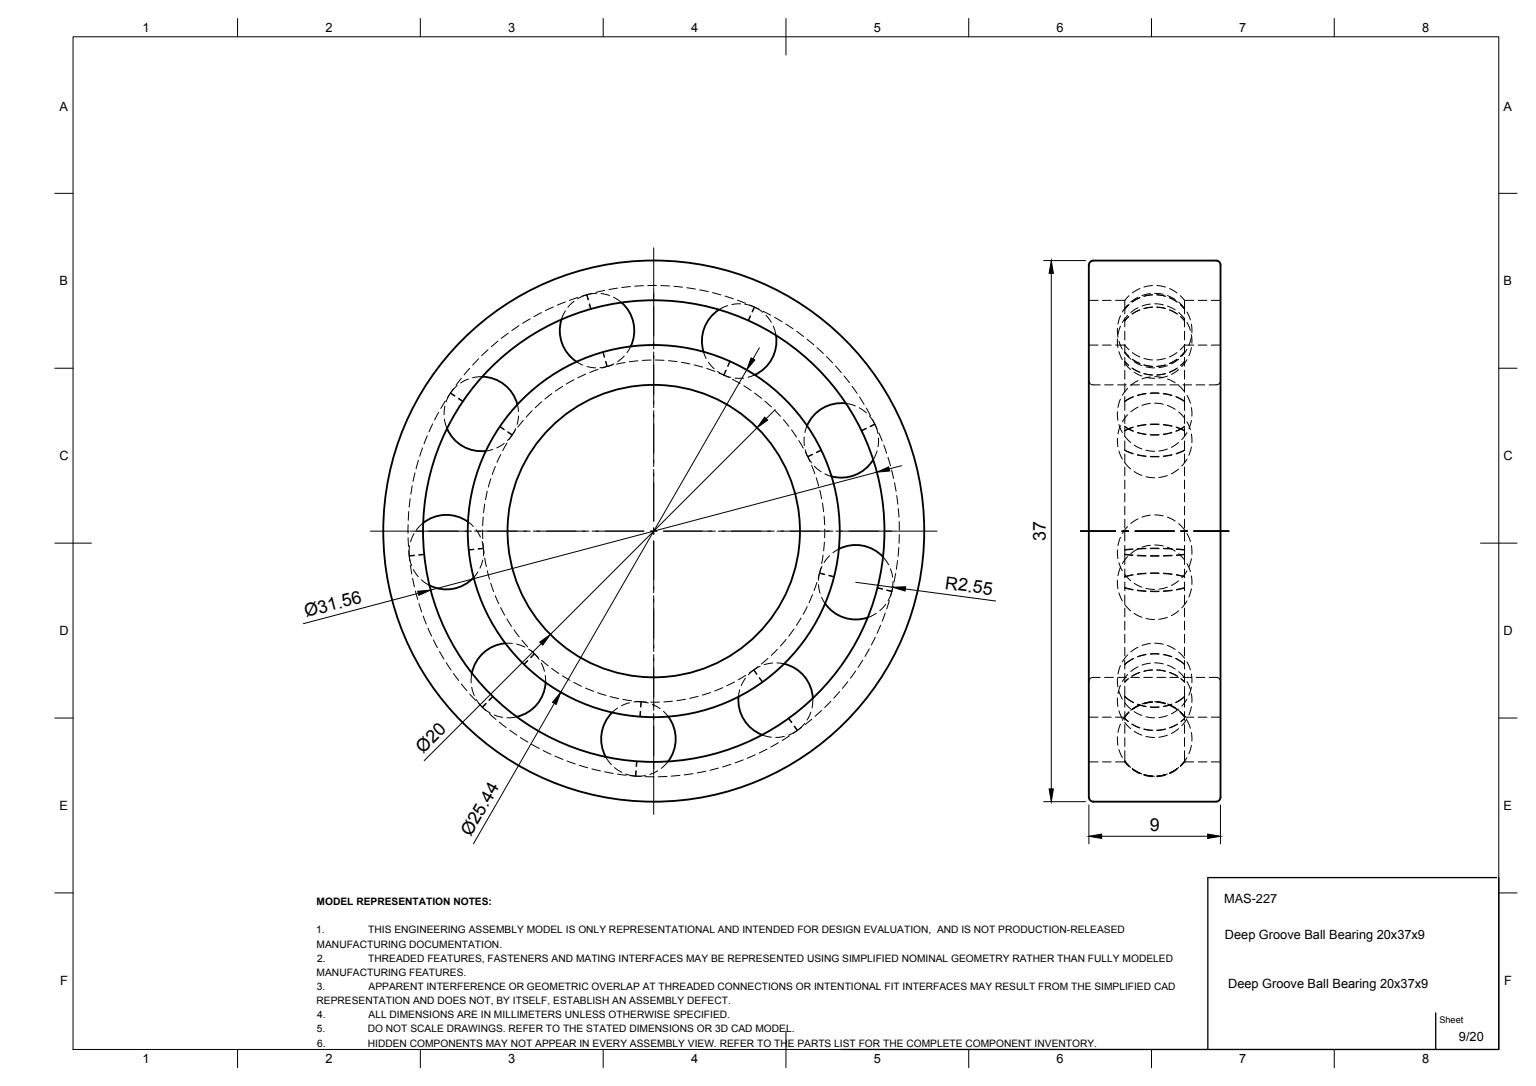
ISO-10303-21;
HEADER;
FILE_DESCRIPTION (('STEP AP214'),
    '1' );
FILE_NAME ( 'Deep Groove Ball Bearing 20x37x9.step', '2026-10-06T08:24:41', ( '' ), ( '' ), 'STEP AP214', 'Unspecified', '' );
FILE_SCHEMA (( 'AUTOMOTIVE_DESIGN' ));
ENDSEC;
DATA;
#3=CARTESIAN_POINT ( 'NONE',  ( -0.4535326485287288212, 0.08054850140359781641, 0.1903859677775356918 ) ) ;
#22=ORIENTED_EDGE ( 'NONE', *, *, #12287, .T. ) ;
#27=ORIENTED_EDGE ( 'NONE', *, *, #23684, .F. ) ;
#29=ORIENTED_EDGE ( 'NONE', *, *, #17755, .F. ) ;
#40=CARTESIAN_POINT ( 'NONE',  ( -2.184900367198595585E-17, 0.6212598425196850238, 0.2574827755769818483 ) ) ;
#60=CARTESIAN_POINT ( 'NONE',  ( -0.4335958738490826581, -0.2505647196907692664, 0.09684793308443542803 ) ) ;
#63=ADVANCED_FACE ( 'NONE', ( #7520 ), #26320, .F. ) ;
#85=ORIENTED_EDGE ( 'NONE', *, *, #20703, .F. ) ;
#95=CARTESIAN_POINT ( 'NONE',  ( 0.1709077104829875848, -0.4707213777573787672, 0.09684874903502814492 ) ) ;
#98=CARTESIAN_POINT ( 'NONE',  ( -0.4055118110236220486, 4.966087413865251393E-17, 0.3543307086614173040 ) ) ;
#129=EDGE_CURVE ( 'NONE', #7282, #11900, #2406, .T. ) ;
#130=TOROIDAL_SURFACE ( 'NONE', #25799, 0.5610236220472440971, 0.1003937007874015908 ) ;
#131=DIRECTION ( 'NONE',  ( 0.000000000000000000, 0.000000000000000000, -1.000000000000000000 ) ) ;
#139=DIRECTION ( 'NONE',  ( 0.000000000000000000, 0.000000000000000000, 1.000000000000000000 ) ) ;
#140=ORIENTED_EDGE ( 'NONE', *, *, #5854, .T. ) ;
#145=ORIENTED_EDGE ( 'NONE', *, *, #17289, .F. ) ;
#146=CARTESIAN_POINT ( 'NONE',  ( -2.183966630091013010E-17, 0.6212598425196852459, 0.09684793308443542803 ) ) ;
#160=DIRECTION ( 'NONE',  ( 0.000000000000000000, 0.000000000000000000, 1.000000000000000000 ) ) ;
#168=CARTESIAN_POINT ( 'NONE',  ( -0.2120693917185543231, -0.5839438448129543602, 0.09684874924366436433 ) ) ;
#180=ORIENTED_EDGE ( 'NONE', *, *, #22193, .F. ) ;
#184=CARTESIAN_POINT ( 'NONE',  ( 0.4932478747986535628, 0.08657132889677619791, 0.09684874903502814492 ) ) ;
#195=CARTESIAN_POINT ( 'NONE',  ( 0.000000000000000000, 0.000000000000000000, -3.278217716535432842E-17 ) ) ;
#198=CARTESIAN_POINT ( 'NONE',  ( -0.1709077104829878069, -0.4707213777573787672, 0.09684874903502814492 ) ) ;
#204=CIRCLE ( 'NONE', #17722, 0.6212598425196850238 ) ;
#210=CIRCLE ( 'NONE', #27230, 0.6212598425196850238 ) ;
#220=CARTESIAN_POINT ( 'NONE',  ( 0.000000000000000000, 0.000000000000000000, 0.1771653543307086520 ) ) ;
#221=EDGE_LOOP ( 'NONE', ( #12338, #6881, #25054, #27642 ) ) ;
#225=CIRCLE ( 'NONE', #16892, 0.5007874015748031704 ) ;
#233=EDGE_CURVE ( 'NONE', #14152, #23049, #22735, .T. ) ;
#248=CARTESIAN_POINT ( 'NONE',  ( 0.3998447049182889956, 0.4754871227240441423, 0.2574803149606298969 ) ) ;
#261=CARTESIAN_POINT ( 'NONE',  ( 0.2965233727166233790, 0.3524965443697388734, 0.1771653543307087630 ) ) ;
#274=ORIENTED_EDGE ( 'NONE', *, *, #6413, .T. ) ;
#279=DIRECTION ( 'NONE',  ( 0.000000000000000000, 1.000000000000000000, 0.000000000000000000 ) ) ;
#290=VERTEX_POINT ( 'NONE', #22923 ) ;
#300=ADVANCED_FACE ( 'NONE', ( #3258 ), #20928, .T. ) ;
#316=ORIENTED_EDGE ( 'NONE', *, *, #13974, .F. ) ;
#318=ORIENTED_EDGE ( 'NONE', *, *, #26206, .F. ) ;
#323=CARTESIAN_POINT ( 'NONE',  ( -0.4126915023524561632, -0.2375990495015092296, 0.2330651858026694390 ) ) ;
#325=CARTESIAN_POINT ( 'NONE',  ( -0.1716509673353403542, -0.4704508543867079173, 0.09684874903502814492 ) ) ;
#327=CARTESIAN_POINT ( 'NONE',  ( 0.5692936381926190226, -0.3294684677443725507, 0.2081850588275903358 ) ) ;
#328=FACE_OUTER_BOUND ( 'NONE', #1258, .T. ) ;
#342=CARTESIAN_POINT ( 'NONE',  ( -0.4333973147258542991, -0.2509079296564011852, 0.09685039370078740717 ) ) ;
#344=ADVANCED_FACE ( 'NONE', ( #1581, #10184 ), #10334, .T. ) ;
#354=CARTESIAN_POINT ( 'NONE',  ( 0.1718374205099799101, -0.4703827404237102550, 0.09685039370078740717 ) ) ;
#377=LINE ( 'NONE', #8956, #9112 ) ;
#393=DIRECTION ( 'NONE',  ( 0.6427876096865396960, 0.7660444431189776804, -0.000000000000000000 ) ) ;
#407=ORIENTED_EDGE ( 'NONE', *, *, #26451, .F. ) ;
#424=CARTESIAN_POINT ( 'NONE',  ( -0.3991696156513551141, 0.4760540497243913594, 0.09684793308443542803 ) ) ;
#437=EDGE_LOOP ( 'NONE', ( #11123, #6651, #25287, #3751, #12023, #11943, #16300, #8034, #5039, #15886, #22940, #20148, #24795, #15480 ) ) ;
#442=ORIENTED_EDGE ( 'NONE', *, *, #8042, .F. ) ;
#448=DIRECTION ( 'NONE',  ( 0.000000000000000000, 1.000000000000000000, 0.000000000000000000 ) ) ;
#450=DIRECTION ( 'NONE',  ( 0.000000000000000000, 0.000000000000000000, 1.000000000000000000 ) ) ;
#454=DIRECTION ( 'NONE',  ( -0.9396926207859082059, 0.3420201433256690460, 0.000000000000000000 ) ) ;
#466=ORIENTED_EDGE ( 'NONE', *, *, #18480, .T. ) ;
#471=DIRECTION ( 'NONE',  ( -0.9848077530122080203, 0.1736481776669311083, 0.000000000000000000 ) ) ;
#473=DIRECTION ( 'NONE',  ( 0.000000000000000000, 0.000000000000000000, 1.000000000000000000 ) ) ;
#474=CARTESIAN_POINT ( 'NONE',  ( 0.1710938124795997883, -0.4706537664821763833, 0.09684793308443542803 ) ) ;
#478=VERTEX_POINT ( 'NONE', #6529 ) ;
#488=ORIENTED_EDGE ( 'NONE', *, *, #21767, .T. ) ;
#505=CARTESIAN_POINT ( 'NONE',  ( 0.6512499169092683671, 0.1155267097728963771, 0.1926811207759472899 ) ) ;
#512=ORIENTED_EDGE ( 'NONE', *, *, #14893, .F. ) ;
#547=CARTESIAN_POINT ( 'NONE',  ( -0.4210617728863489950, -0.2437762437896736079, 0.2467937633087636806 ) ) ;
#553=CARTESIAN_POINT ( 'NONE',  ( -0.2956505864974144360, 0.3532288989643737054, 0.1903859677777559323 ) ) ;
#564=AXIS2_PLACEMENT_3D ( 'NONE', #14105, #3204, #1666 ) ;
#566=DIRECTION ( 'NONE',  ( 0.000000000000000000, 0.000000000000000000, 1.000000000000000000 ) ) ;
#568=CARTESIAN_POINT ( 'NONE',  ( -0.1669561253487713837, -0.4569961989594632512, 0.2467937633337932146 ) ) ;
#580=ADVANCED_FACE ( 'NONE', ( #26282 ), #25912, .F. ) ;
#588=EDGE_CURVE ( 'NONE', #1674, #11878, #12352, .T. ) ;
#590=DIRECTION ( 'NONE',  ( -1.000000000000000000, 1.224646799147346305E-16, 0.000000000000000000 ) ) ;
#595=ADVANCED_FACE ( 'NONE', ( #719 ), #17319, .T. ) ;
#621=CARTESIAN_POINT ( 'NONE',  ( -0.5383572925356228112, -0.3100567972183445042, 0.2574803149606298969 ) ) ;
#625=FACE_OUTER_BOUND ( 'NONE', #9890, .T. ) ;
#639=DIRECTION ( 'NONE',  ( 0.000000000000000000, 0.000000000000000000, 1.000000000000000000 ) ) ;
#640=ORIENTED_EDGE ( 'NONE', *, *, #8614, .T. ) ;
#659=CARTESIAN_POINT ( 'NONE',  ( 0.6119360453657125554, 0.1072290460171897442, 0.09685039370078740717 ) ) ;
#692=ORIENTED_EDGE ( 'NONE', *, *, #26206, .T. ) ;
#693=CARTESIAN_POINT ( 'NONE',  ( 0.000000000000000000, 0.000000000000000000, 0.3425196850393700809 ) ) ;
#702=CARTESIAN_POINT ( 'NONE',  ( -0.0005939837304750000086, 0.5007870493127504208, 0.2574803149606298969 ) ) ;
#705=EDGE_CURVE ( 'NONE', #13715, #9472, #19846, .T. ) ;
#719=FACE_OUTER_BOUND ( 'NONE', #2456, .T. ) ;
#730=VERTEX_POINT ( 'NONE', #18485 ) ;
#731=DIRECTION ( 'NONE',  ( 0.000000000000000000, 1.000000000000000000, 0.000000000000000000 ) ) ;
#746=EDGE_CURVE ( 'NONE', #25825, #26393, #21042, .T. ) ;
#747=CARTESIAN_POINT ( 'NONE',  ( 0.6117833106356003192, 0.1080972763116094665, 0.2574827755769819038 ) ) ;
#753=TOROIDAL_SURFACE ( 'NONE', #16532, 0.7165354330708662012, 0.01181102362204724393 ) ;
#760=B_SPLINE_CURVE_WITH_KNOTS ( 'NONE', 3,
 ( #11709, #11429, #14120, #13834, #3353, #22726 ),
 .UNSPECIFIED., .F., .F.,
 ( 4, 2, 4 ),
 ( 0.9031406754215589583, 0.9046454396443730506, 0.9061502038671870318 ),
 .UNSPECIFIED. ) ;
#761=CARTESIAN_POINT ( 'NONE',  ( -7.608238775805210269E-17, -0.6212598425196850238, 0.3059055118110236560 ) ) ;
#765=EDGE_CURVE ( 'NONE', #26553, #20265, #18689, .T. ) ;
#769=CARTESIAN_POINT ( 'NONE',  ( -0.4931105264837953306, 0.08735026989778622852, 0.09684874903502814492 ) ) ;
#772=CARTESIAN_POINT ( 'NONE',  ( 0.000000000000000000, 0.000000000000000000, 0.3425196850393700809 ) ) ;
#776=DIRECTION ( 'NONE',  ( 0.000000000000000000, 0.000000000000000000, 1.000000000000000000 ) ) ;
#777=MECHANICAL_DESIGN_GEOMETRIC_PRESENTATION_REPRESENTATION('',(#15229),#16556);
#798=VERTEX_POINT ( 'NONE', #6495 ) ;
#811=DIRECTION ( 'NONE',  ( 0.000000000000000000, 1.000000000000000000, 0.000000000000000000 ) ) ;
#818=CARTESIAN_POINT ( 'NONE',  ( 0.6117062799105531523, 0.1085321106658064944, 0.2574803149606298969 ) ) ;
#829=CARTESIAN_POINT ( 'NONE',  ( 0.4121125639445893385, -0.2386018002037871011, 0.1212655228849990885 ) ) ;
#832=CARTESIAN_POINT ( 'NONE',  ( 0.2118615749922464486, -0.5840192333899535404, 0.2574803149606298969 ) ) ;
#833=VERTEX_POINT ( 'NONE', #19057 ) ;
#852=DIRECTION ( 'NONE',  ( 0.000000000000000000, 1.000000000000000000, 0.000000000000000000 ) ) ;
#882=CARTESIAN_POINT ( 'NONE',  ( -0.2255758929758618081, -0.6217623271429643106, 0.1616495878894404215 ) ) ;
#887=CARTESIAN_POINT ( 'NONE',  ( -0.4931450244001936989, 0.08715529520342381320, 0.2574827755769819038 ) ) ;
#897=FACE_OUTER_BOUND ( 'NONE', #27032, .T. ) ;
#900=CARTESIAN_POINT ( 'NONE',  ( -0.3998447049182095037, 0.4754871227241110332, 0.2574803149606298969 ) ) ;
#941=ORIENTED_EDGE ( 'NONE', *, *, #17711, .F. ) ;
#958=CARTESIAN_POINT ( 'NONE',  ( 0.000000000000000000, 0.000000000000000000, -3.278217716535432842E-17 ) ) ;
#969=EDGE_CURVE ( 'NONE', #16082, #26393, #16448, .T. ) ;
#973=CARTESIAN_POINT ( 'NONE',  ( 0.2243259791921815294, -0.6183223858027685482, 0.2081850588255441115 ) ) ;
#980=ORIENTED_EDGE ( 'NONE', *, *, #22815, .T. ) ;
#982=ORIENTED_EDGE ( 'NONE', *, *, #7627, .T. ) ;
#1008=CARTESIAN_POINT ( 'NONE',  ( -0.3223547283257516272, 0.3832433309296771617, 0.09685039370078740717 ) ) ;
#1013=ORIENTED_EDGE ( 'NONE', *, *, #10554, .F. ) ;
#1015=DIRECTION ( 'NONE',  ( 1.000000000000000000, 0.000000000000000000, 0.000000000000000000 ) ) ;
#1022=ORIENTED_EDGE ( 'NONE', *, *, #21337, .F. ) ;
#1026=ADVANCED_FACE ( 'NONE', ( #5184 ), #7886, .F. ) ;
#1040=CARTESIAN_POINT ( 'NONE',  ( 0.1707210962531913734, -0.4707890492249701131, 0.2574803149606298969 ) ) ;
#1042=CARTESIAN_POINT ( 'NONE',  ( 0.3998447049182889956, 0.4754871227240441423, 0.2574803149606298969 ) ) ;
#1044=DIRECTION ( 'NONE',  ( 1.000000000000000000, 0.000000000000000000, 0.000000000000000000 ) ) ;
#1057=DIRECTION ( 'NONE',  ( 0.000000000000000000, 0.000000000000000000, -1.000000000000000000 ) ) ;
#1074=DIRECTION ( 'NONE',  ( 0.000000000000000000, 0.000000000000000000, 1.000000000000000000 ) ) ;
#1079=ORIENTED_EDGE ( 'NONE', *, *, #19204, .T. ) ;
#1101=EDGE_CURVE ( 'NONE', #17070, #17929, #9204, .T. ) ;
#1110=DIRECTION ( 'NONE',  ( -0.8660254037844385966, -0.5000000000000002220, 0.000000000000000000 ) ) ;
#1116=CARTESIAN_POINT ( 'NONE',  ( 0.1589886963209722337, -0.4351482077926094871, 0.1494804571181609920 ) ) ;
#1126=EDGE_LOOP ( 'NONE', ( #5710, #17595 ) ) ;
#1132=EDGE_CURVE ( 'NONE', #24679, #11735, #20131, .T. ) ;
#1165=VERTEX_POINT ( 'NONE', #5771 ) ;
#1167=ORIENTED_EDGE ( 'NONE', *, *, #24794, .F. ) ;
#1175=ORIENTED_EDGE ( 'NONE', *, *, #10870, .F. ) ;
#1180=FACE_OUTER_BOUND ( 'NONE', #1413, .T. ) ;
#1185=ORIENTED_EDGE ( 'NONE', *, *, #7200, .F. ) ;
#1193=ORIENTED_EDGE ( 'NONE', *, *, #9457, .F. ) ;
#1195=DIRECTION ( 'NONE',  ( 0.000000000000000000, 0.000000000000000000, 1.000000000000000000 ) ) ;
#1205=VECTOR ( 'NONE', #24148, 39.37007874015748143 ) ;
#1224=EDGE_LOOP ( 'NONE', ( #22539, #14658 ) ) ;
#1229=B_SPLINE_CURVE_WITH_KNOTS ( 'NONE', 3,
 ( #14885, #198, #17116, #11030, #325, #8767 ),
 .UNSPECIFIED., .F., .F.,
 ( 4, 2, 4 ),
 ( 0.3000437156586439613, 0.3015484798814569989, 0.3030532441042709801 ),
 .UNSPECIFIED. ) ;
#1240=CARTESIAN_POINT ( 'NONE',  ( 0.4535326485287339282, 0.08054850140356757671, 0.1771653543307084855 ) ) ;
#1252=ORIENTED_EDGE ( 'NONE', *, *, #21408, .T. ) ;
#1253=CARTESIAN_POINT ( 'NONE',  ( 0.2255758929755326547, -0.6217623271420399389, 0.1616495878830931654 ) ) ;
#1258=EDGE_LOOP ( 'NONE', ( #23878, #2968, #26517, #23453 ) ) ;
#1271=CIRCLE ( 'NONE', #26511, 0.7165354330708662012 ) ;
#1272=CARTESIAN_POINT ( 'NONE',  ( 0.000000000000000000, 0.000000000000000000, 0.3059055118110236560 ) ) ;
#1280=EDGE_CURVE ( 'NONE', #12816, #3515, #3825, .T. ) ;
#1282=CARTESIAN_POINT ( 'NONE',  ( 0.2956505864974371400, 0.3532288989643546651, 0.1771653543307085410 ) ) ;
#1285=ADVANCED_FACE ( 'NONE', ( #11976, #20594 ), #16633, .T. ) ;
#1293=CARTESIAN_POINT ( 'NONE',  ( -0.2161007281675216829, -0.5956855348323873978, 0.2481708550952000381 ) ) ;
#1302=CARTESIAN_POINT ( 'NONE',  ( 0.000000000000000000, 0.000000000000000000, 0.1771653543307086520 ) ) ;
#1315=AXIS2_PLACEMENT_3D ( 'NONE', #21292, #9201, #22211 ) ;
#1319=ORIENTED_EDGE ( 'NONE', *, *, #129, .F. ) ;
#1345=DIRECTION ( 'NONE',  ( 0.000000000000000000, 0.000000000000000000, 1.000000000000000000 ) ) ;
#1360=CARTESIAN_POINT ( 'NONE',  ( 0.1918813796216842782, -0.5271897577243779276, 0.1771653543307086520 ) ) ;
#1369=CARTESIAN_POINT ( 'NONE',  ( 0.4535326485287340947, 0.08054850140356764610, 0.1639447408599974121 ) ) ;
#1374=AXIS2_PLACEMENT_3D ( 'NONE', #3401, #5409, #20799 ) ;
#1393=CARTESIAN_POINT ( 'NONE',  ( 0.2126900928101059240, -0.5837180524351401889, 0.09684793308443542803 ) ) ;
#1395=CARTESIAN_POINT ( 'NONE',  ( 0.1718374205099799101, -0.4703827404237102550, 0.2574803149606298969 ) ) ;
#1401=CARTESIAN_POINT ( 'NONE',  ( 0.2131049448084480213, -0.5835666837866708700, 0.2574803149606298969 ) ) ;
#1408=B_SPLINE_CURVE_WITH_KNOTS ( 'NONE', 3,
 ( #24286, #18184, #26974, #22591, #568, #5506 ),
 .UNSPECIFIED., .F., .F.,
 ( 4, 2, 4 ),
 ( 0.5000000000000000000, 0.7500000000000000000, 1.000000000000000000 ),
 .UNSPECIFIED. ) ;
#1412=DIRECTION ( 'NONE',  ( 1.000000000000000000, 0.000000000000000000, 0.000000000000000000 ) ) ;
#1413=EDGE_LOOP ( 'NONE', ( #8075, #11194 ) ) ;
#1417=FACE_OUTER_BOUND ( 'NONE', #16441, .T. ) ;
#1422=CARTESIAN_POINT ( 'NONE',  ( 0.000000000000000000, 0.000000000000000000, 0.1771653543307086520 ) ) ;
#1423=VECTOR ( 'NONE', #6934, 39.37007874015748143 ) ;
#1429=CARTESIAN_POINT ( 'NONE',  ( -0.0001974756197918548992, 0.5007874015748031704, 0.09684793308443542803 ) ) ;
#1441=ORIENTED_EDGE ( 'NONE', *, *, #12607, .F. ) ;
#1468=B_SPLINE_CURVE_WITH_KNOTS ( 'NONE', 3,
 ( #6685, #13435, #24188, #6962, #11059, #6547 ),
 .UNSPECIFIED., .F., .F.,
 ( 4, 2, 4 ),
 ( 0.3108507187342960387, 0.3125269569790670166, 0.3142031952238389936 ),
 .UNSPECIFIED. ) ;
#1482=EDGE_LOOP ( 'NONE', ( #17416, #8893 ) ) ;
#1483=DIRECTION ( 'NONE',  ( 0.000000000000000000, 1.000000000000000000, 0.000000000000000000 ) ) ;
#1525=CARTESIAN_POINT ( 'NONE',  ( -0.4078284417470132150, 0.4849914877844211936, 0.1061598535650708358 ) ) ;
#1528=AXIS2_PLACEMENT_3D ( 'NONE', #24169, #20201, #454 ) ;
#1545=CARTESIAN_POINT ( 'NONE',  ( 0.000000000000000000, 0.000000000000000000, 0.09685039370078740717 ) ) ;
#1551=CARTESIAN_POINT ( 'NONE',  ( 0.2120693917185216271, -0.5839438448129662396, 0.2574819594177531479 ) ) ;
#1555=CARTESIAN_POINT ( 'NONE',  ( 0.3122922550358837035, 0.3730863453234792848, 0.1075369453527844910 ) ) ;
#1576=CIRCLE ( 'NONE', #6546, 0.6212598425196850238 ) ;
#1581=FACE_OUTER_BOUND ( 'NONE', #21227, .T. ) ;
#1583=CARTESIAN_POINT ( 'NONE',  ( -0.4055118110236220486, 4.966087413865251393E-17, 0.3425196850393700809 ) ) ;
#1594=ADVANCED_FACE ( 'NONE', ( #13215, #2743 ), #5009, .T. ) ;
#1615=SHAPE_REPRESENTATION ( 'Deep Groove Ball Bearing 20x37x9', ( #11588 ), #25599 ) ;
#1617=EDGE_LOOP ( 'NONE', ( #26636, #12625 ) ) ;
#1649=DIRECTION ( 'NONE',  ( 0.000000000000000000, 0.000000000000000000, 1.000000000000000000 ) ) ;
#1654=FACE_OUTER_BOUND ( 'NONE', #1126, .T. ) ;
#1666=DIRECTION ( 'NONE',  ( 0.000000000000000000, -1.000000000000000000, 0.000000000000000000 ) ) ;
#1674=VERTEX_POINT ( 'NONE', #2446 ) ;
#1691=CARTESIAN_POINT ( 'NONE',  ( 1.456051859513969730E-17, 0.5007874015748032814, 0.2574827755769819038 ) ) ;
#1695=CIRCLE ( 'NONE', #12060, 0.6212598425196850238 ) ;
#1698=ORIENTED_EDGE ( 'NONE', *, *, #10194, .F. ) ;
#1704=ORIENTED_EDGE ( 'NONE', *, *, #19694, .F. ) ;
#1713=ORIENTED_EDGE ( 'NONE', *, *, #14644, .F. ) ;
#1721=DIRECTION ( 'NONE',  ( 0.3420201433256691570, -0.9396926207859082059, 0.000000000000000000 ) ) ;
#1739=ORIENTED_EDGE ( 'NONE', *, *, #13974, .T. ) ;
#1741=AXIS2_PLACEMENT_3D ( 'NONE', #19071, #4646, #2125 ) ;
#1775=EDGE_LOOP ( 'NONE', ( #13680, #19313, #6854, #316, #10783, #6020, #16688, #25651, #23336, #23483, #140, #14286, #18043 ) ) ;
#1781=DIRECTION ( 'NONE',  ( 0.000000000000000000, 0.000000000000000000, -1.000000000000000000 ) ) ;
#1782=CARTESIAN_POINT ( 'NONE',  ( 0.6117062799105453808, 0.1085321106658576895, 0.09685039370078740717 ) ) ;
#1783=DIRECTION ( 'NONE',  ( 0.000000000000000000, -1.000000000000000000, 0.000000000000000000 ) ) ;
#1784=ADVANCED_FACE ( 'NONE', ( #7526, #1180 ), #25038, .T. ) ;
#1795=ORIENTED_EDGE ( 'NONE', *, *, #27521, .F. ) ;
#1804=VERTEX_POINT ( 'NONE', #3547 ) ;
#1816=AXIS2_PLACEMENT_3D ( 'NONE', #10489, #25619, #21244 ) ;
#1822=CIRCLE ( 'NONE', #7231, 0.1003956692913385990 ) ;
#1823=B_SPLINE_CURVE_WITH_KNOTS ( 'NONE', 3,
 ( #1040, #3129, #9631, #18236, #26446, #7110 ),
 .UNSPECIFIED., .F., .F.,
 ( 4, 2, 4 ),
 ( 0.9031406754215579591, 0.9046454396443710522, 0.9061502038671850334 ),
 .UNSPECIFIED. ) ;
#1843=DIRECTION ( 'NONE',  ( 0.000000000000000000, 0.000000000000000000, 1.000000000000000000 ) ) ;
#1852=CARTESIAN_POINT ( 'NONE',  ( 0.4690668203917182089, 0.08212126673940543797, 0.2330651858111663088 ) ) ;
#1862=CARTESIAN_POINT ( 'NONE',  ( 0.0005696707463081691122, 0.4606295689977897845, 0.1903859677794648431 ) ) ;
#1869=VERTEX_POINT ( 'NONE', #16006 ) ;
#1870=ORIENTED_EDGE ( 'NONE', *, *, #765, .F. ) ;
#1871=AXIS2_PLACEMENT_3D ( 'NONE', #22035, #21385, #11297 ) ;
#1885=CARTESIAN_POINT ( 'NONE',  ( -6.132876883919029269E-17, -0.5007874015748031704, 0.3059055118110236560 ) ) ;
#1894=DIRECTION ( 'NONE',  ( 0.000000000000000000, -1.000000000000000000, 0.000000000000000000 ) ) ;
#1896=ORIENTED_EDGE ( 'NONE', *, *, #10087, .F. ) ;
#1911=EDGE_CURVE ( 'NONE', #1674, #11878, #18256, .T. ) ;
#1958=TOROIDAL_SURFACE ( 'NONE', #5096, 0.5610236220472440971, 0.1003937007874015908 ) ;
#1964=CIRCLE ( 'NONE', #24961, 0.4055118110236220486 ) ;
#1970=FACE_BOUND ( 'NONE', #21845, .T. ) ;
#1977=AXIS2_PLACEMENT_3D ( 'NONE', #6220, #4092, #12279 ) ;
#1987=CARTESIAN_POINT ( 'NONE',  ( -0.4932821129636645874, 0.08637579872942342807, 0.2574803149606298969 ) ) ;
#1988=CARTESIAN_POINT ( 'NONE',  ( -0.3998447049182496382, 0.4754871227240771714, 0.09685039370078740717 ) ) ;
#2008=VERTEX_POINT ( 'NONE', #16083 ) ;
#2031=DIRECTION ( 'NONE',  ( 1.224646799147353207E-16, 1.000000000000000000, -0.000000000000000000 ) ) ;
#2052=CARTESIAN_POINT ( 'NONE',  ( -0.5572789388083557727, -0.3225230913466954896, 0.1183902030405236949 ) ) ;
#2057=CARTESIAN_POINT ( 'NONE',  ( 0.3606190329934327310, 0.4297690281277732338, 0.1771653543307086520 ) ) ;
#2070=EDGE_CURVE ( 'NONE', #17929, #16979, #5269, .T. ) ;
#2089=DIRECTION ( 'NONE',  ( 0.000000000000000000, 1.000000000000000000, 0.000000000000000000 ) ) ;
#2094=DIRECTION ( 'NONE',  ( 0.000000000000000000, 0.000000000000000000, 1.000000000000000000 ) ) ;
#2119=B_SPLINE_CURVE_WITH_KNOTS ( 'NONE', 3,
 ( #16214, #7741, #12392, #13956, #22567, #20730 ),
 .UNSPECIFIED., .F., .F.,
 ( 4, 2, 4 ),
 ( 0.000000000000000000, 0.2500000000000000000, 0.5000000000000000000 ),
 .UNSPECIFIED. ) ;
#2121=AXIS2_PLACEMENT_3D ( 'NONE', #25906, #19405, #13042 ) ;
#2123=CARTESIAN_POINT ( 'NONE',  ( 0.4931105264837953306, 0.08735026989778582607, 0.09684874903502814492 ) ) ;
#2125=DIRECTION ( 'NONE',  ( -0.1736481776669299426, 0.9848077530122081313, 0.000000000000000000 ) ) ;
#2138=DIRECTION ( 'NONE',  ( 0.000000000000000000, 0.000000000000000000, 1.000000000000000000 ) ) ;
#2146=ORIENTED_EDGE ( 'NONE', *, *, #14178, .T. ) ;
#2150=EDGE_LOOP ( 'NONE', ( #2358, #2146 ) ) ;
#2156=DIRECTION ( 'NONE',  ( 0.000000000000000000, 0.000000000000000000, 1.000000000000000000 ) ) ;
#2159=B_SPLINE_CURVE_WITH_KNOTS ( 'NONE', 3,
 ( #26441, #3, #7107, #13452, #8569, #15725 ),
 .UNSPECIFIED., .F., .F.,
 ( 4, 2, 4 ),
 ( 0.5000000000000000000, 0.7500000000000000000, 1.000000000000000000 ),
 .UNSPECIFIED. ) ;
#2176=AXIS2_PLACEMENT_3D ( 'NONE', #25126, #20756, #23318 ) ;
#2188=ORIENTED_EDGE ( 'NONE', *, *, #7551, .T. ) ;
#2193=B_SPLINE_CURVE_WITH_KNOTS ( 'NONE', 3,
 ( #1042, #15735, #20099, #14032, #26319, #20526, #15859, #17831, #13599, #5265 ),
 .UNSPECIFIED., .F., .F.,
 ( 4, 2, 2, 2, 4 ),
 ( 0.000000000000000000, 0.2500000000000000000, 0.5000000000000000000, 0.7500000000000000000, 1.000000000000000000 ),
 .UNSPECIFIED. ) ;
#2215=ORIENTED_EDGE ( 'NONE', *, *, #25261, .F. ) ;
#2232=CARTESIAN_POINT ( 'NONE',  ( 0.3992017438595159562, -0.2298214351608004746, 0.1771653543307084855 ) ) ;
#2233=EDGE_CURVE ( 'NONE', #20284, #17070, #24466, .T. ) ;
#2234=CIRCLE ( 'NONE', #23000, 0.5007874015748031704 ) ;
#2235=DIRECTION ( 'NONE',  ( 1.000000000000000000, 0.000000000000000000, 0.000000000000000000 ) ) ;
#2248=ORIENTED_EDGE ( 'NONE', *, *, #17807, .F. ) ;
#2261=DIRECTION ( 'NONE',  ( 0.000000000000000000, 0.000000000000000000, 1.000000000000000000 ) ) ;
#2269=CARTESIAN_POINT ( 'NONE',  ( 0.000000000000000000, 0.000000000000000000, 0.2574803149606298969 ) ) ;
#2273=AXIS2_PLACEMENT_3D ( 'NONE', #26937, #2903, #20015 ) ;
#2288=B_SPLINE_CURVE_WITH_KNOTS ( 'NONE', 3,
 ( #13606, #26190, #6848, #13061, #6989, #248 ),
 .UNSPECIFIED., .F., .F.,
 ( 4, 2, 4 ),
 ( 0.9359046326922999537, 0.9375808709372039917, 0.9392571091821070306 ),
 .UNSPECIFIED. ) ;
#2290=AXIS2_PLACEMENT_3D ( 'NONE', #20850, #5604, #16474 ) ;
#2292=CARTESIAN_POINT ( 'NONE',  ( 0.4133615125893445597, 0.4936731914951132949, 0.1183902030404491851 ) ) ;
#2304=AXIS2_PLACEMENT_3D ( 'NONE', #2730, #11361, #7124 ) ;
#2311=CARTESIAN_POINT ( 'NONE',  ( -0.0006615832605804723319, 0.6212594902576319411, 0.2574803149606298969 ) ) ;
#2330=CARTESIAN_POINT ( 'NONE',  ( 0.000000000000000000, 0.000000000000000000, 0.1771653543307086520 ) ) ;
#2331=EDGE_LOOP ( 'NONE', ( #5331, #5512, #8568, #18130 ) ) ;
#2353=ORIENTED_EDGE ( 'NONE', *, *, #25470, .F. ) ;
#2358=ORIENTED_EDGE ( 'NONE', *, *, #12014, .F. ) ;
#2396=CARTESIAN_POINT ( 'NONE',  ( 0.000000000000000000, 0.000000000000000000, 0.1771653543307086520 ) ) ;
#2397=CARTESIAN_POINT ( 'NONE',  ( 0.2973550541884159570, 0.3552623538120610602, 0.2048502514842716338 ) ) ;
#2401=DIRECTION ( 'NONE',  ( 0.000000000000000000, 0.000000000000000000, 1.000000000000000000 ) ) ;
#2403=CARTESIAN_POINT ( 'NONE',  ( -0.0005939837304750000086, 0.5007870493127504208, 0.09685039370078740717 ) ) ;
#2406=CIRCLE ( 'NONE', #5580, 0.1003956692913385851 ) ;
#2419=EDGE_CURVE ( 'NONE', #290, #27249, #26173, .T. ) ;
#2421=DIRECTION ( 'NONE',  ( 0.000000000000000000, 0.000000000000000000, 1.000000000000000000 ) ) ;
#2427=EDGE_LOOP ( 'NONE', ( #10019, #27204, #13449, #9599 ) ) ;
#2442=CARTESIAN_POINT ( 'NONE',  ( 0.000000000000000000, 0.000000000000000000, -3.278217716535432842E-17 ) ) ;
#2446=CARTESIAN_POINT ( 'NONE',  ( -0.1918813796216842782, -0.5271897577243779276, 0.07676968503937006694 ) ) ;
#2454=TOROIDAL_SURFACE ( 'NONE', #4688, 0.4055118110236220486, 0.01181102362204724393 ) ;
#2456=EDGE_LOOP ( 'NONE', ( #3138, #14628, #3299, #24249, #2555 ) ) ;
#2472=B_SPLINE_CURVE_WITH_KNOTS ( 'NONE', 3,
 ( #24519, #14078, #22838, #12092, #5167, #3034 ),
 .UNSPECIFIED., .F., .F.,
 ( 4, 2, 4 ),
 ( 0.5000000000000000000, 0.7500000000000000000, 1.000000000000000000 ),
 .UNSPECIFIED. ) ;
#2479=B_SPLINE_CURVE_WITH_KNOTS ( 'NONE', 3,
 ( #21751, #553, #23880, #10867, #19763, #9277 ),
 .UNSPECIFIED., .F., .F.,
 ( 4, 2, 4 ),
 ( 0.5000000000000000000, 0.7500000000000000000, 1.000000000000000000 ),
 .UNSPECIFIED. ) ;
#2509=ORIENTED_EDGE ( 'NONE', *, *, #15940, .T. ) ;
#2515=CARTESIAN_POINT ( 'NONE',  ( 0.000000000000000000, 0.000000000000000000, 0.09685039370078740717 ) ) ;
#2534=CIRCLE ( 'NONE', #18307, 0.6212598425196850238 ) ;
#2540=AXIS2_PLACEMENT_3D ( 'NONE', #18666, #12049, #20945 ) ;
#2555=ORIENTED_EDGE ( 'NONE', *, *, #16773, .T. ) ;
#2581=TOROIDAL_SURFACE ( 'NONE', #9808, 0.5610236220472440971, 0.1003937007874015908 ) ;
#2588=DIRECTION ( 'NONE',  ( 0.000000000000000000, 0.000000000000000000, 1.000000000000000000 ) ) ;
#2602=CARTESIAN_POINT ( 'NONE',  ( 0.6339803004464725777, 0.1124719464480360975, 0.1183902030413380158 ) ) ;
#2620=CARTESIAN_POINT ( 'NONE',  ( -0.6512499169089656093, 0.1155267097728523984, 0.1616495878834900424 ) ) ;
#2622=CARTESIAN_POINT ( 'NONE',  ( 0.000000000000000000, 0.000000000000000000, 0.2574803149606298969 ) ) ;
#2628=VERTEX_POINT ( 'NONE', #21147 ) ;
#2637=CARTESIAN_POINT ( 'NONE',  ( 0.000000000000000000, 0.000000000000000000, 0.1771653543307086520 ) ) ;
#2640=CARTESIAN_POINT ( 'NONE',  ( -6.132876883919029269E-17, -0.5007874015748031704, 0.2574803149606298969 ) ) ;
#2646=EDGE_CURVE ( 'NONE', #11007, #6574, #1695, .T. ) ;
#2651=AXIS2_PLACEMENT_3D ( 'NONE', #5903, #1649, #10254 ) ;
#2652=DIRECTION ( 'NONE',  ( 0.000000000000000000, 0.000000000000000000, 1.000000000000000000 ) ) ;
#2667=CARTESIAN_POINT ( 'NONE',  ( 0.3988311005573134116, 0.4763376377694984454, 0.09685039370078740717 ) ) ;
#2675=ADVANCED_FACE ( 'NONE', ( #18435, #27363 ), #8013, .T. ) ;
#2681=DIRECTION ( 'NONE',  ( 0.000000000000000000, 1.000000000000000000, 0.000000000000000000 ) ) ;
#2683=TOROIDAL_SURFACE ( 'NONE', #4951, 0.5610236220472440971, 0.1003937007874015908 ) ;
#2684=TOROIDAL_SURFACE ( 'NONE', #9004, 0.5610236220472440971, 0.1003937007874015908 ) ;
#2688=CARTESIAN_POINT ( 'NONE',  ( 0.000000000000000000, 0.000000000000000000, 0.09685039370078740717 ) ) ;
#2691=CARTESIAN_POINT ( 'NONE',  ( -0.4690668203699855932, 0.08212126673558327317, 0.1212655228837342947 ) ) ;
#2702=VERTEX_POINT ( 'NONE', #7731 ) ;
#2717=CARTESIAN_POINT ( 'NONE',  ( 0.4858607088160724063, -0.2805118110236220486, 0.1771653543307086520 ) ) ;
#2730=CARTESIAN_POINT ( 'NONE',  ( -0.4858607088160732390, -0.2805118110236220486, 0.1771653543307086520 ) ) ;
#2740=CIRCLE ( 'NONE', #24408, 0.3937007874015748254 ) ;
#2743=FACE_BOUND ( 'NONE', #15245, .T. ) ;
#2747=VERTEX_POINT ( 'NONE', #19151 ) ;
#2775=CARTESIAN_POINT ( 'NONE',  ( 0.000000000000000000, 0.000000000000000000, 0.09685039370078740717 ) ) ;
#2781=EDGE_LOOP ( 'NONE', ( #16201, #23225, #21886, #15230 ) ) ;
#2789=ORIENTED_EDGE ( 'NONE', *, *, #5062, .T. ) ;
#2797=CARTESIAN_POINT ( 'NONE',  ( -0.1580799066051627177, -0.4326553680327468454, 0.1771653543307088186 ) ) ;
#2805=CARTESIAN_POINT ( 'NONE',  ( 0.7165354330708662012, 0.000000000000000000, -3.278217716535432842E-17 ) ) ;
#2814=ORIENTED_EDGE ( 'NONE', *, *, #17711, .T. ) ;
#2817=ORIENTED_EDGE ( 'NONE', *, *, #21955, .T. ) ;
#2823=DIRECTION ( 'NONE',  ( 0.000000000000000000, 0.000000000000000000, 1.000000000000000000 ) ) ;
#2829=DIRECTION ( 'NONE',  ( 0.9848077530122081313, 0.1736481776669299981, -0.000000000000000000 ) ) ;
#2833=CARTESIAN_POINT ( 'NONE',  ( -0.1707210962531915677, -0.4707890492249701131, 0.2574803149606298969 ) ) ;
#2847=CARTESIAN_POINT ( 'NONE',  ( -0.5699748819080105999, -0.3282885190149778531, 0.2081850588304353933 ) ) ;
#2855=AXIS2_PLACEMENT_3D ( 'NONE', #1583, #18370, #12041 ) ;
#2858=CARTESIAN_POINT ( 'NONE',  ( 0.5699748819079695217, -0.3282885190149665844, 0.2081850588305529104 ) ) ;
#2890=AXIS2_PLACEMENT_3D ( 'NONE', #2515, #2652, #11278 ) ;
#2896=B_SPLINE_CURVE_WITH_KNOTS ( 'NONE', 3,
 ( #11826, #20446, #3333, #16216, #20160, #17882 ),
 .UNSPECIFIED., .F., .F.,
 ( 4, 2, 4 ),
 ( 0.3000437156586439613, 0.3015484798814569989, 0.3030532441042709801 ),
 .UNSPECIFIED. ) ;
#2899=DIRECTION ( 'NONE',  ( 0.000000000000000000, 0.000000000000000000, 1.000000000000000000 ) ) ;
#2902=EDGE_CURVE ( 'NONE', #16455, #17891, #6228, .T. ) ;
#2903=DIRECTION ( 'NONE',  ( 0.000000000000000000, 0.000000000000000000, 1.000000000000000000 ) ) ;
#2920=VERTEX_POINT ( 'NONE', #21971 ) ;
#2939=CARTESIAN_POINT ( 'NONE',  ( -0.0005789383928838939082, 0.4762008496974535765, 0.2330651857776422364 ) ) ;
#2943=CYLINDRICAL_SURFACE ( 'NONE', #8673, 0.5007874015748031704 ) ;
#2951=AXIS2_PLACEMENT_3D ( 'NONE', #17165, #15609, #13060 ) ;
#2952=CARTESIAN_POINT ( 'NONE',  ( 0.4216473063928389275, -0.2427620699807058191, 0.1075369453624760163 ) ) ;
#2968=ORIENTED_EDGE ( 'NONE', *, *, #21663, .F. ) ;
#2985=CARTESIAN_POINT ( 'NONE',  ( 0.0005696707463077370576, 0.4606295689977898400, 0.1771653543307089018 ) ) ;
#2986=CARTESIAN_POINT ( 'NONE',  ( -0.5491102354215389170, -0.3162573801172571808, 0.2481708550950527947 ) ) ;
#2987=EDGE_CURVE ( 'NONE', #5913, #9216, #24812, .T. ) ;
#3034=CARTESIAN_POINT ( 'NONE',  ( -0.3223547283257516272, 0.3832433309296771617, 0.09685039370078740717 ) ) ;
#3075=DIRECTION ( 'NONE',  ( 0.000000000000000000, -1.000000000000000000, 0.000000000000000000 ) ) ;
#3079=FACE_OUTER_BOUND ( 'NONE', #14199, .T. ) ;
#3082=CARTESIAN_POINT ( 'NONE',  ( -0.4222761783109335032, 0.5043089796502874256, 0.2081850588267502022 ) ) ;
#3083=AXIS2_PLACEMENT_3D ( 'NONE', #23793, #9069, #4438 ) ;
#3086=ORIENTED_EDGE ( 'NONE', *, *, #17207, .F. ) ;
#3093=B_SPLINE_CURVE_WITH_KNOTS ( 'NONE', 3,
 ( #702, #22308, #2939, #14710, #14845, #8185 ),
 .UNSPECIFIED., .F., .F.,
 ( 4, 2, 4 ),
 ( 0.000000000000000000, 0.2500000000000000000, 0.5000000000000000000 ),
 .UNSPECIFIED. ) ;
#3129=CARTESIAN_POINT ( 'NONE',  ( 0.1709077104829875848, -0.4707213777573787672, 0.2574819596263889787 ) ) ;
#3130=FACE_OUTER_BOUND ( 'NONE', #2150, .T. ) ;
#3131=CARTESIAN_POINT ( 'NONE',  ( 0.3222028160008074682, 0.3833711078595924970, 0.2574819596263889787 ) ) ;
#3135=DIRECTION ( 'NONE',  ( 0.000000000000000000, 0.000000000000000000, 1.000000000000000000 ) ) ;
#3138=ORIENTED_EDGE ( 'NONE', *, *, #23236, .F. ) ;
#3141=ORIENTED_EDGE ( 'NONE', *, *, #21514, .F. ) ;
#3150=AXIS2_PLACEMENT_3D ( 'NONE', #6820, #24869, #11879 ) ;
#3151=DIRECTION ( 'NONE',  ( 0.000000000000000000, 0.000000000000000000, 1.000000000000000000 ) ) ;
#3152=EDGE_CURVE ( 'NONE', #6711, #11971, #24912, .T. ) ;
#3160=VERTEX_POINT ( 'NONE', #11502 ) ;
#3167=B_SPLINE_CURVE_WITH_KNOTS ( 'NONE', 3,
 ( #10551, #16646, #19174, #17064, #23013, #27385 ),
 .UNSPECIFIED., .F., .F.,
 ( 4, 2, 4 ),
 ( 0.000000000000000000, 0.2500000000000000000, 0.5000000000000000000 ),
 .UNSPECIFIED. ) ;
#3182=CIRCLE ( 'NONE', #20802, 0.1003956692913386267 ) ;
#3189=CARTESIAN_POINT ( 'NONE',  ( 0.6241612306998541859, 0.1093779649449431318, 0.1061598535669114746 ) ) ;
#3192=CARTESIAN_POINT ( 'NONE',  ( -0.5379168165870276130, -0.3108204284649299098, 0.09684793308443542803 ) ) ;
#3204=DIRECTION ( 'NONE',  ( 0.000000000000000000, 0.000000000000000000, -1.000000000000000000 ) ) ;
#3214=ORIENTED_EDGE ( 'NONE', *, *, #15264, .T. ) ;
#3256=CARTESIAN_POINT ( 'NONE',  ( 0.000000000000000000, 0.000000000000000000, 0.1771653543307086520 ) ) ;
#3258=FACE_OUTER_BOUND ( 'NONE', #14398, .T. ) ;
#3273=FACE_BOUND ( 'NONE', #23803, .T. ) ;
#3277=CIRCLE ( 'NONE', #19540, 0.7283464566929134243 ) ;
#3282=CARTESIAN_POINT ( 'NONE',  ( 0.5383572925355968319, -0.3100567972183901899, 0.09685039370078740717 ) ) ;
#3284=DIRECTION ( 'NONE',  ( 0.000000000000000000, 0.000000000000000000, 1.000000000000000000 ) ) ;
#3299=ORIENTED_EDGE ( 'NONE', *, *, #24840, .T. ) ;
#3309=EDGE_CURVE ( 'NONE', #11845, #25113, #17201, .T. ) ;
#3333=CARTESIAN_POINT ( 'NONE',  ( 0.3217486617182078734, 0.3837523410419874659, 0.09684793308443542803 ) ) ;
#3336=DIRECTION ( 'NONE',  ( 0.000000000000000000, 0.000000000000000000, -1.000000000000000000 ) ) ;
#3347=ORIENTED_EDGE ( 'NONE', *, *, #8429, .F. ) ;
#3349=CIRCLE ( 'NONE', #14675, 0.1003956692913385990 ) ;
#3353=CARTESIAN_POINT ( 'NONE',  ( 0.4931105264837953306, 0.08735026989778603423, 0.2574819596263889787 ) ) ;
#3386=CARTESIAN_POINT ( 'NONE',  ( -0.1579154690106709391, -0.4355388305871915056, 0.1494804571213769195 ) ) ;
#3399=DIRECTION ( 'NONE',  ( 0.000000000000000000, 0.000000000000000000, 1.000000000000000000 ) ) ;
#3401=CARTESIAN_POINT ( 'NONE',  ( 0.000000000000000000, 0.5610236220472440971, 0.3543307086614173040 ) ) ;
#3413=ORIENTED_EDGE ( 'NONE', *, *, #20354, .F. ) ;
#3418=CARTESIAN_POINT ( 'NONE',  ( 0.5383572925355708527, -0.3100567972184350429, 0.2574803149606298969 ) ) ;
#3428=EDGE_CURVE ( 'NONE', #14935, #24679, #9414, .T. ) ;
#3453=AXIS2_PLACEMENT_3D ( 'NONE', #15418, #24005, #19767 ) ;
#3454=CIRCLE ( 'NONE', #17881, 0.5007874015748031704 ) ;
#3464=EDGE_CURVE ( 'NONE', #14369, #27683, #17089, .T. ) ;
#3475=CARTESIAN_POINT ( 'NONE',  ( 0.0006737210091392942029, 0.6438792636745043207, 0.2359405056220706121 ) ) ;
#3492=ORIENTED_EDGE ( 'NONE', *, *, #27512, .T. ) ;
#3502=CARTESIAN_POINT ( 'NONE',  ( 0.000000000000000000, 0.000000000000000000, 0.2574803149606298969 ) ) ;
#3503=CARTESIAN_POINT ( 'NONE',  ( 0.5376957092749645728, -0.3112026930392428614, 0.09685039370078740717 ) ) ;
#3506=EDGE_CURVE ( 'NONE', #18857, #16353, #27007, .T. ) ;
#3511=CARTESIAN_POINT ( 'NONE',  ( 0.2965233727166233790, 0.3524965443697388734, 0.1771653543307087630 ) ) ;
#3515=VERTEX_POINT ( 'NONE', #4291 ) ;
#3523=EDGE_LOOP ( 'NONE', ( #19442, #21347, #13019, #12962 ) ) ;
#3529=CARTESIAN_POINT ( 'NONE',  ( -0.2195865873856400752, -0.6052790189082013494, 0.2359405056219452124 ) ) ;
#3532=CARTESIAN_POINT ( 'NONE',  ( -0.0003954787107570692452, 0.5007872847596378518, 0.09684874903502814492 ) ) ;
#3533=ORIENTED_EDGE ( 'NONE', *, *, #10907, .T. ) ;
#3547=CARTESIAN_POINT ( 'NONE',  ( 0.5376957092749645728, -0.3112026930392428614, 0.09685039370078740717 ) ) ;
#3576=ADVANCED_FACE ( 'NONE', ( #23240 ), #25659, .F. ) ;
#3593=EDGE_CURVE ( 'NONE', #15868, #17285, #8064, .T. ) ;
#3601=CARTESIAN_POINT ( 'NONE',  ( 0.000000000000000000, 0.000000000000000000, 0.01181102362204724393 ) ) ;
#3612=AXIS2_PLACEMENT_3D ( 'NONE', #17620, #13651, #26234 ) ;
#3614=ORIENTED_EDGE ( 'NONE', *, *, #8978, .T. ) ;
#3617=CARTESIAN_POINT ( 'NONE',  ( -0.5382469622846938195, -0.3102483656526051625, 0.09684874924366436433 ) ) ;
#3650=UNCERTAINTY_MEASURE_WITH_UNIT (LENGTH_MEASURE( 1.000000000000000082E-05 ), #13265, 'distance_accuracy_value', 'NONE') ;
#3665=DIRECTION ( 'NONE',  ( 0.000000000000000000, 0.000000000000000000, 1.000000000000000000 ) ) ;
#3668=CARTESIAN_POINT ( 'NONE',  ( -0.3217486617182078734, 0.3837523410419874659, 0.09684793308443542803 ) ) ;
#3670=CARTESIAN_POINT ( 'NONE',  ( 0.000000000000000000, 0.000000000000000000, 0.1771653543307086520 ) ) ;
#3675=DIRECTION ( 'NONE',  ( 0.000000000000000000, 0.000000000000000000, 1.000000000000000000 ) ) ;
#3690=EDGE_LOOP ( 'NONE', ( #8728, #7708, #10424, #22 ) ) ;
#3694=EDGE_CURVE ( 'NONE', #21183, #11904, #22054, .T. ) ;
#3713=DIRECTION ( 'NONE',  ( 1.000000000000000000, 0.000000000000000000, 0.000000000000000000 ) ) ;
#3732=ORIENTED_EDGE ( 'NONE', *, *, #9757, .T. ) ;
#3737=CARTESIAN_POINT ( 'NONE',  ( 0.000000000000000000, 0.000000000000000000, 0.04842519685039370358 ) ) ;
#3742=EDGE_CURVE ( 'NONE', #12816, #21648, #26115, .T. ) ;
#3751=ORIENTED_EDGE ( 'NONE', *, *, #2987, .T. ) ;
#3753=DIRECTION ( 'NONE',  ( 0.000000000000000000, 1.000000000000000000, 0.000000000000000000 ) ) ;
#3783=CARTESIAN_POINT ( 'NONE',  ( -0.4233199042353229524, 0.5034331896078060309, 0.1461456498253434766 ) ) ;
#3793=ORIENTED_EDGE ( 'NONE', *, *, #8211, .T. ) ;
#3802=CARTESIAN_POINT ( 'NONE',  ( 0.4339912984563291110, -0.2498791196563492356, 0.2574803149606298969 ) ) ;
#3805=CARTESIAN_POINT ( 'NONE',  ( -0.3223547283257516272, 0.3832433309296771617, 0.2574803149606298969 ) ) ;
#3818=VERTEX_POINT ( 'NONE', #7877 ) ;
#3825=CIRCLE ( 'NONE', #21438, 0.1003937007874015908 ) ;
#3828=EDGE_CURVE ( 'NONE', #12846, #24919, #25958, .T. ) ;
#3829=DIRECTION ( 'NONE',  ( 0.000000000000000000, 0.000000000000000000, 1.000000000000000000 ) ) ;
#3832=ADVANCED_FACE ( 'NONE', ( #16625 ), #8079, .F. ) ;
#3833=CIRCLE ( 'NONE', #14234, 0.6212598425196850238 ) ;
#3836=CARTESIAN_POINT ( 'NONE',  ( -0.5525004126151165096, 0.09742072959660473541, 0.1771653543307086520 ) ) ;
#3867=EDGE_CURVE ( 'NONE', #9254, #22901, #4394, .T. ) ;
#3888=CARTESIAN_POINT ( 'NONE',  ( 0.4121125639456494349, -0.2386018002044008601, 0.2330651857782768399 ) ) ;
#3896=CARTESIAN_POINT ( 'NONE',  ( 0.000000000000000000, 0.5610236220472440971, 0.1771653543307086520 ) ) ;
#3902=EDGE_CURVE ( 'NONE', #11779, #25825, #25203, .T. ) ;
#3915=CIRCLE ( 'NONE', #4809, 0.4055118110236220486 ) ;
#3921=ORIENTED_EDGE ( 'NONE', *, *, #15046, .F. ) ;
#3924=VERTEX_POINT ( 'NONE', #11198 ) ;
#3929=ORIENTED_EDGE ( 'NONE', *, *, #15264, .F. ) ;
#3957=ADVANCED_FACE ( 'NONE', ( #26181 ), #21610, .F. ) ;
#3965=CARTESIAN_POINT ( 'NONE',  ( 0.1918813796216842782, -0.5271897577243779276, 0.07676968503937006694 ) ) ;
#3966=ORIENTED_EDGE ( 'NONE', *, *, #19654, .T. ) ;
#3976=CARTESIAN_POINT ( 'NONE',  ( 0.4563437505065279232, 0.07988585396532887906, 0.2048502514943769115 ) ) ;
#3980=AXIS2_PLACEMENT_3D ( 'NONE', #17523, #27720, #8365 ) ;
#4007=VERTEX_POINT ( 'NONE', #2805 ) ;
#4015=ORIENTED_EDGE ( 'NONE', *, *, #12014, .T. ) ;
#4057=TOROIDAL_SURFACE ( 'NONE', #8129, 0.5610236220472440971, 0.1003937007874015908 ) ;
#4083=AXIS2_PLACEMENT_3D ( 'NONE', #25482, #23381, #12622 ) ;
#4087=EDGE_LOOP ( 'NONE', ( #18164, #26808, #16298, #25957, #3141, #10241 ) ) ;
#4092=DIRECTION ( 'NONE',  ( 0.000000000000000000, 0.000000000000000000, 1.000000000000000000 ) ) ;
#4096=EDGE_CURVE ( 'NONE', #798, #12635, #2896, .T. ) ;
#4101=DIRECTION ( 'NONE',  ( 0.9396926207859082059, -0.3420201433256691015, 0.000000000000000000 ) ) ;
#4106=DIRECTION ( 'NONE',  ( 0.000000000000000000, -1.000000000000000000, 0.000000000000000000 ) ) ;
#4145=CARTESIAN_POINT ( 'NONE',  ( 0.000000000000000000, 0.000000000000000000, 0.1771653543307086520 ) ) ;
#4148=CARTESIAN_POINT ( 'NONE',  ( 0.4222761783102037536, 0.5043089796494211186, 0.2081850588299743177 ) ) ;
#4181=CARTESIAN_POINT ( 'NONE',  ( -0.5724622793728307846, -0.3313001865995510720, 0.1926811207742144816 ) ) ;
#4208=CARTESIAN_POINT ( 'NONE',  ( -0.6239291699148459269, 0.1106940470466721976, 0.1061598535656959191 ) ) ;
#4223=ADVANCED_FACE ( 'NONE', ( #5906, #1654 ), #16631, .T. ) ;
#4231=AXIS2_PLACEMENT_3D ( 'NONE', #5476, #27092, #20158 ) ;
#4233=AXIS2_PLACEMENT_3D ( 'NONE', #6903, #18150, #22011 ) ;
#4245=CARTESIAN_POINT ( 'NONE',  ( 0.000000000000000000, 0.000000000000000000, 0.3425196850393700809 ) ) ;
#4246=ORIENTED_EDGE ( 'NONE', *, *, #21408, .F. ) ;
#4252=ORIENTED_EDGE ( 'NONE', *, *, #14545, .F. ) ;
#4253=CARTESIAN_POINT ( 'NONE',  ( -0.4333973147258542991, -0.2509079296564011852, 0.09685039370078740717 ) ) ;
#4265=CARTESIAN_POINT ( 'NONE',  ( 0.6478824768876890738, 0.1135474080048673312, 0.2081850588311874306 ) ) ;
#4276=ADVANCED_FACE ( 'NONE', ( #18446 ), #20262, .F. ) ;
#4282=ORIENTED_EDGE ( 'NONE', *, *, #26906, .F. ) ;
#4288=CARTESIAN_POINT ( 'NONE',  ( -0.4563437504957677526, 0.07988585396341746359, 0.1494804572056230296 ) ) ;
#4289=CARTESIAN_POINT ( 'NONE',  ( -0.3991696156513685478, 0.4760540497243803681, 0.2574827755769819038 ) ) ;
#4291=CARTESIAN_POINT ( 'NONE',  ( 0.5007874015748030594, 0.000000000000000000, 0.09685039370078740717 ) ) ;
#4314=ORIENTED_EDGE ( 'NONE', *, *, #22479, .F. ) ;
#4328=CARTESIAN_POINT ( 'NONE',  ( 0.000000000000000000, 0.000000000000000000, -3.278217716535432842E-17 ) ) ;
#4341=ORIENTED_EDGE ( 'NONE', *, *, #14178, .F. ) ;
#4348=CARTESIAN_POINT ( 'NONE',  ( -0.2965233727166468602, 0.3524965443697189449, 0.1903859677771958248 ) ) ;
#4354=CARTESIAN_POINT ( 'NONE',  ( 0.6117062799105453808, 0.1085321106658576895, 0.09685039370078740717 ) ) ;
#4377=EDGE_CURVE ( 'NONE', #10201, #16332, #26831, .T. ) ;
#4389=CARTESIAN_POINT ( 'NONE',  ( -0.4334967711386992772, -0.2507361369899905879, 0.09684874903502814492 ) ) ;
#4394=B_SPLINE_CURVE_WITH_KNOTS ( 'NONE', 3,
 ( #9844, #23133, #3475, #27514, #14677, #18870, #6045, #14244, #27652, #12104 ),
 .UNSPECIFIED., .F., .F.,
 ( 4, 2, 2, 2, 4 ),
 ( 0.000000000000000000, 0.2500000000000000000, 0.5000000000000000000, 0.7500000000000000000, 1.000000000000000000 ),
 .UNSPECIFIED. ) ;
#4398=CARTESIAN_POINT ( 'NONE',  ( 0.1570092758121685861, -0.4330450457732857306, 0.1639447408159873665 ) ) ;
#4412=EDGE_CURVE ( 'NONE', #16082, #27489, #1229, .T. ) ;
#4438=DIRECTION ( 'NONE',  ( 0.000000000000000000, 1.000000000000000000, 0.000000000000000000 ) ) ;
#4443=DIRECTION ( 'NONE',  ( 0.7660444431189777914, -0.6427876096865396960, 0.000000000000000000 ) ) ;
#4448=EDGE_CURVE ( 'NONE', #5352, #13907, #21185, .T. ) ;
#4467=EDGE_CURVE ( 'NONE', #11052, #11455, #23463, .T. ) ;
#4468=CARTESIAN_POINT ( 'NONE',  ( -0.6119360453657027854, 0.1072290460172413279, 0.2574803149606298969 ) ) ;
#4481=EDGE_LOOP ( 'NONE', ( #14759, #8403, #7371, #12289 ) ) ;
#4494=ORIENTED_EDGE ( 'NONE', *, *, #14386, .T. ) ;
#4503=EDGE_CURVE ( 'NONE', #17070, #10201, #15405, .T. ) ;
#4534=CARTESIAN_POINT ( 'NONE',  ( 0.1579154690111878589, -0.4355388305886193634, 0.1494804571160150142 ) ) ;
#4537=CARTESIAN_POINT ( 'NONE',  ( 0.5724622793732239145, -0.3313001865997644568, 0.1926811207713212126 ) ) ;
#4541=EDGE_CURVE ( 'NONE', #20920, #26710, #22131, .T. ) ;
#4558=CARTESIAN_POINT ( 'NONE',  ( 0.3988311005572732215, 0.4763376377695315300, 0.2574803149606298969 ) ) ;
#4561=CARTESIAN_POINT ( 'NONE',  ( 0.000000000000000000, 0.000000000000000000, 0.09685039370078740717 ) ) ;
#4585=CARTESIAN_POINT ( 'NONE',  ( -0.3992017438595018564, -0.2298214351608254269, 0.1771653543307087630 ) ) ;
#4601=EDGE_LOOP ( 'NONE', ( #8593, #488, #3966, #15163 ) ) ;
#4602=AXIS2_PLACEMENT_3D ( 'NONE', #20757, #18330, #16510 ) ;
#4610=ORIENTED_EDGE ( 'NONE', *, *, #17812, .F. ) ;
#4617=ORIENTED_EDGE ( 'NONE', *, *, #15636, .T. ) ;
#4626=VECTOR ( 'NONE', #24210, 39.37007874015748143 ) ;
#4638=LENGTH_MEASURE_WITH_UNIT ( LENGTH_MEASURE( 0.02539999999999999897 ), #11144 ) ;
#4646=DIRECTION ( 'NONE',  ( 0.9848077530122082424, 0.1736481776669299149, -0.000000000000000000 ) ) ;
#4649=VERTEX_POINT ( 'NONE', #20650 ) ;
#4663=B_SPLINE_CURVE_WITH_KNOTS ( 'NONE', 3,
 ( #16020, #20111, #12056, #20675, #769, #9358 ),
 .UNSPECIFIED., .F., .F.,
 ( 4, 2, 4 ),
 ( 0.3000437156586439613, 0.3015484798814579981, 0.3030532441042709801 ),
 .UNSPECIFIED. ) ;
#4681=FACE_OUTER_BOUND ( 'NONE', #8261, .T. ) ;
#4685=CARTESIAN_POINT ( 'NONE',  ( -0.5525004126151165096, 0.09742072959660473541, 0.1771653543307086520 ) ) ;
#4688=AXIS2_PLACEMENT_3D ( 'NONE', #8241, #10061, #18815 ) ;
#4699=CARTESIAN_POINT ( 'NONE',  ( 3.644242538420618632E-18, 0.5007874015748032814, 0.09684793308443545579 ) ) ;
#4700=SPHERICAL_SURFACE ( 'NONE', #5819, 0.1003956692913385851 ) ;
#4708=EDGE_CURVE ( 'NONE', #22917, #18857, #12599, .T. ) ;
#4730=ORIENTED_EDGE ( 'NONE', *, *, #20377, .F. ) ;
#4737=CARTESIAN_POINT ( 'NONE',  ( -0.3214446924536846772, 0.3840069416942866742, 0.2574803149606298969 ) ) ;
#4739=VERTEX_POINT ( 'NONE', #19510 ) ;
#4749=ADVANCED_FACE ( 'NONE', ( #328 ), #25632, .F. ) ;
#4769=DIRECTION ( 'NONE',  ( 0.000000000000000000, 0.000000000000000000, 1.000000000000000000 ) ) ;
#4781=LINE ( 'NONE', #15419, #1205 ) ;
#4809=AXIS2_PLACEMENT_3D ( 'NONE', #17963, #24618, #5276 ) ;
#4810=EDGE_CURVE ( 'NONE', #10058, #27798, #16685, .T. ) ;
#4819=CARTESIAN_POINT ( 'NONE',  ( -0.4537304931026617250, 0.07942646906834203990, 0.1639447408816315788 ) ) ;
#4821=CARTESIAN_POINT ( 'NONE',  ( 0.000000000000000000, 0.000000000000000000, 0.3425196850393700809 ) ) ;
#4830=EDGE_CURVE ( 'NONE', #6451, #14713, #16029, .T. ) ;
#4845=CARTESIAN_POINT ( 'NONE',  ( -0.1570092758121683640, -0.4330450457732857306, 0.1903859678374740794 ) ) ;
#4851=VERTEX_POINT ( 'NONE', #7302 ) ;
#4855=FACE_BOUND ( 'NONE', #27837, .T. ) ;
#4862=AXIS2_PLACEMENT_3D ( 'NONE', #3502, #24984, #18472 ) ;
#4864=CARTESIAN_POINT ( 'NONE',  ( 0.7165354330708662012, 0.000000000000000000, 0.3425196850393700809 ) ) ;
#4908=AXIS2_PLACEMENT_3D ( 'NONE', #2269, #450, #25873 ) ;
#4911=CARTESIAN_POINT ( 'NONE',  ( -0.3986320731132245165, -0.2308081338369633306, 0.1903859677991110999 ) ) ;
#4914=CARTESIAN_POINT ( 'NONE',  ( 0.4333973147258542991, -0.2509079296564015737, 0.09685039370078740717 ) ) ;
#4916=CARTESIAN_POINT ( 'NONE',  ( 0.4932821129636645874, 0.08637579872942321990, 0.09685039370078740717 ) ) ;
#4918=EDGE_LOOP ( 'NONE', ( #26016, #24345, #19720, #17060, #16164, #5271, #13298, #19391, #25253, #5442, #2817, #17351, #27201, #9989 ) ) ;
#4920=ADVANCED_FACE ( 'NONE', ( #20372 ), #16615, .F. ) ;
#4943=ORIENTED_EDGE ( 'NONE', *, *, #21983, .T. ) ;
#4944=DIRECTION ( 'NONE',  ( 1.000000000000000000, 0.000000000000000000, 0.000000000000000000 ) ) ;
#4951=AXIS2_PLACEMENT_3D ( 'NONE', #19111, #8108, #17139 ) ;
#4955=AXIS2_PLACEMENT_3D ( 'NONE', #7217, #19941, #5237 ) ;
#4965=AXIS2_PLACEMENT_3D ( 'NONE', #19468, #160, #811 ) ;
#4984=CARTESIAN_POINT ( 'NONE',  ( 0.1918813796216842782, -0.5271897577243779276, 0.1771653543307086520 ) ) ;
#4993=CARTESIAN_POINT ( 'NONE',  ( 0.000000000000000000, 0.000000000000000000, 0.3425196850393700809 ) ) ;
#5000=CARTESIAN_POINT ( 'NONE',  ( 3.644242538420618632E-18, 0.5007874015748032814, 0.09684793308443545579 ) ) ;
#5009=SPHERICAL_SURFACE ( 'NONE', #24579, 0.1003956692913385851 ) ;
#5018=CARTESIAN_POINT ( 'NONE',  ( -2.183966630091013010E-17, 0.6212598425196852459, 0.09684793308443542803 ) ) ;
#5021=ORIENTED_EDGE ( 'NONE', *, *, #17755, .T. ) ;
#5029=EDGE_LOOP ( 'NONE', ( #12681, #25468, #3492, #692 ) ) ;
#5030=ORIENTED_EDGE ( 'NONE', *, *, #12576, .T. ) ;
#5039=ORIENTED_EDGE ( 'NONE', *, *, #22013, .F. ) ;
#5043=CIRCLE ( 'NONE', #19028, 0.6212598425196850238 ) ;
#5056=EDGE_CURVE ( 'NONE', #14228, #10058, #13664, .T. ) ;
#5062=EDGE_CURVE ( 'NONE', #24230, #3515, #24729, .T. ) ;
#5064=DIRECTION ( 'NONE',  ( 0.000000000000000000, 0.000000000000000000, 1.000000000000000000 ) ) ;
#5067=CARTESIAN_POINT ( 'NONE',  ( 0.000000000000000000, 0.000000000000000000, 0.3425196850393700809 ) ) ;
#5068=CARTESIAN_POINT ( 'NONE',  ( -0.3992017438595021339, -0.2298214351608249550, 0.1903859677995012600 ) ) ;
#5096=AXIS2_PLACEMENT_3D ( 'NONE', #26432, #24876, #22626 ) ;
#5105=CARTESIAN_POINT ( 'NONE',  ( 0.6119360453657027854, 0.1072290460172409393, 0.2574803149606298969 ) ) ;
#5112=DIRECTION ( 'NONE',  ( 0.8660254037844385966, -0.5000000000000000000, 0.000000000000000000 ) ) ;
#5117=AXIS2_PLACEMENT_3D ( 'NONE', #22324, #19928, #7207 ) ;
#5139=CARTESIAN_POINT ( 'NONE',  ( -7.608238775805210269E-17, -0.6212598425196850238, 0.09685039370078740717 ) ) ;
#5146=B_SPLINE_CURVE_WITH_KNOTS ( 'NONE', 3,
 ( #1782, #27650, #2602, #17717, #22108, #505, #11228, #13622, #26339, #17848 ),
 .UNSPECIFIED., .F., .F.,
 ( 4, 2, 2, 2, 4 ),
 ( 0.000000000000000000, 0.2500000000000000000, 0.5000000000000000000, 0.7500000000000000000, 1.000000000000000000 ),
 .UNSPECIFIED. ) ;
#5167=CARTESIAN_POINT ( 'NONE',  ( -0.3131893444210941957, 0.3723335979309581600, 0.1075369453644233753 ) ) ;
#5176=CARTESIAN_POINT ( 'NONE',  ( 0.6514872030421683391, 0.1141809932449793924, 0.1616495878895669036 ) ) ;
#5184=FACE_OUTER_BOUND ( 'NONE', #16091, .T. ) ;
#5186=EDGE_CURVE ( 'NONE', #19404, #24230, #14719, .T. ) ;
#5189=AXIS2_PLACEMENT_3D ( 'NONE', #220, #2156, #6541 ) ;
#5215=CIRCLE ( 'NONE', #25540, 0.6212598425196850238 ) ;
#5229=CARTESIAN_POINT ( 'NONE',  ( 0.000000000000000000, 0.000000000000000000, 0.000000000000000000 ) ) ;
#5237=DIRECTION ( 'NONE',  ( 0.000000000000000000, -1.000000000000000000, 0.000000000000000000 ) ) ;
#5265=CARTESIAN_POINT ( 'NONE',  ( 0.3998447049182496382, 0.4754871227240771714, 0.09685039370078740717 ) ) ;
#5269=B_SPLINE_CURVE_WITH_KNOTS ( 'NONE', 3,
 ( #4914, #26253, #829, #13527, #7317, #22432 ),
 .UNSPECIFIED., .F., .F.,
 ( 4, 2, 4 ),
 ( 0.000000000000000000, 0.2500000000000000000, 0.5000000000000000000 ),
 .UNSPECIFIED. ) ;
#5271=ORIENTED_EDGE ( 'NONE', *, *, #9231, .T. ) ;
#5276=DIRECTION ( 'NONE',  ( 0.000000000000000000, -1.000000000000000000, 0.000000000000000000 ) ) ;
#5291=TOROIDAL_SURFACE ( 'NONE', #19744, 0.5610236220472440971, 0.1003937007874015908 ) ;
#5319=FACE_OUTER_BOUND ( 'NONE', #18999, .T. ) ;
#5331=ORIENTED_EDGE ( 'NONE', *, *, #10267, .F. ) ;
#5341=EDGE_LOOP ( 'NONE', ( #21168, #1185, #24144, #3614 ) ) ;
#5347=ORIENTED_EDGE ( 'NONE', *, *, #6996, .F. ) ;
#5352=VERTEX_POINT ( 'NONE', #25425 ) ;
#5356=CARTESIAN_POINT ( 'NONE',  ( 0.000000000000000000, 0.7283464566929134243, 0.01181102362204724393 ) ) ;
#5359=CARTESIAN_POINT ( 'NONE',  ( 0.5378064472801062923, -0.3110113600220468233, 0.09684874924366436433 ) ) ;
#5366=AXIS2_PLACEMENT_3D ( 'NONE', #1302, #7513, #9908 ) ;
#5388=CARTESIAN_POINT ( 'NONE',  ( 0.7283464566929135353, 0.000000000000000000, 0.3425196850393700809 ) ) ;
#5391=CARTESIAN_POINT ( 'NONE',  ( -0.2195865873860579631, -0.6052790189093463225, 0.1183902030410438760 ) ) ;
#5409=DIRECTION ( 'NONE',  ( 0.000000000000000000, 0.000000000000000000, 1.000000000000000000 ) ) ;
#5412=SPHERICAL_SURFACE ( 'NONE', #20826, 0.1003956692913385851 ) ;
#5418=DIRECTION ( 'NONE',  ( 0.9848077530122081313, 0.1736481776669299981, -0.000000000000000000 ) ) ;
#5429=CARTESIAN_POINT ( 'NONE',  ( 0.4858607088160724063, -0.2805118110236220486, 0.2775610236220472093 ) ) ;
#5442=ORIENTED_EDGE ( 'NONE', *, *, #7200, .T. ) ;
#5460=ORIENTED_EDGE ( 'NONE', *, *, #14509, .F. ) ;
#5461=ORIENTED_EDGE ( 'NONE', *, *, #2070, .F. ) ;
#5471=CIRCLE ( 'NONE', #19017, 0.6212598425196850238 ) ;
#5476=CARTESIAN_POINT ( 'NONE',  ( 0.4858607088160724063, -0.2805118110236220486, 0.1771653543307086520 ) ) ;
#5479=DIRECTION ( 'NONE',  ( -0.5000000000000001110, 0.8660254037844384856, 0.000000000000000000 ) ) ;
#5481=CARTESIAN_POINT ( 'NONE',  ( 0.3065394984574514314, 0.3644188803065985249, 0.2330651858034864243 ) ) ;
#5501=EDGE_CURVE ( 'NONE', #2628, #8924, #18353, .T. ) ;
#5506=CARTESIAN_POINT ( 'NONE',  ( -0.1718374205099799101, -0.4703827404237102550, 0.2574803149606298969 ) ) ;
#5512=ORIENTED_EDGE ( 'NONE', *, *, #15471, .T. ) ;
#5518=EDGE_CURVE ( 'NONE', #27249, #6246, #11221, .T. ) ;
#5523=CIRCLE ( 'NONE', #20464, 0.4606299212598425341 ) ;
#5549=DIRECTION ( 'NONE',  ( 1.000000000000000000, 0.000000000000000000, 0.000000000000000000 ) ) ;
#5555=EDGE_LOOP ( 'NONE', ( #8348, #21160, #7773, #25328, #21358, #1713 ) ) ;
#5557=FACE_BOUND ( 'NONE', #11418, .T. ) ;
#5560=VERTEX_POINT ( 'NONE', #16357 ) ;
#5570=CARTESIAN_POINT ( 'NONE',  ( 0.1707210962531913734, -0.4707890492249701131, 0.2574803149606298969 ) ) ;
#5580=AXIS2_PLACEMENT_3D ( 'NONE', #26578, #23829, #22353 ) ;
#5581=ADVANCED_FACE ( 'NONE', ( #7596, #8537 ), #20447, .T. ) ;
#5592=CIRCLE ( 'NONE', #14654, 0.7165354330708662012 ) ;
#5603=CARTESIAN_POINT ( 'NONE',  ( -0.2131049448083992270, -0.5835666837866889667, 0.09685039370078740717 ) ) ;
#5604=DIRECTION ( 'NONE',  ( 0.000000000000000000, 0.000000000000000000, 1.000000000000000000 ) ) ;
#5618=DIRECTION ( 'NONE',  ( 0.000000000000000000, -1.000000000000000000, 0.000000000000000000 ) ) ;
#5662=CARTESIAN_POINT ( 'NONE',  ( 0.3056525133779917636, 0.3651631491557606468, 0.1212655228624319320 ) ) ;
#5663=ORIENTED_EDGE ( 'NONE', *, *, #19218, .T. ) ;
#5667=B_SPLINE_CURVE_WITH_KNOTS ( 'NONE', 3,
 ( #26188, #17698, #21960, #22085, #4845, #21685 ),
 .UNSPECIFIED., .F., .F.,
 ( 4, 2, 4 ),
 ( 0.000000000000000000, 0.2500000000000000000, 0.5000000000000000000 ),
 .UNSPECIFIED. ) ;
#5673=VERTEX_POINT ( 'NONE', #26183 ) ;
#5674=AXIS2_PLACEMENT_3D ( 'NONE', #2622, #7149, #279 ) ;
#5681=ADVANCED_FACE ( 'NONE', ( #9205, #15464 ), #4700, .T. ) ;
#5684=CARTESIAN_POINT ( 'NONE',  ( -0.6119360453657027854, 0.1072290460172413279, 0.2574803149606298969 ) ) ;
#5699=CIRCLE ( 'NONE', #20574, 0.6212598425196850238 ) ;
#5703=CIRCLE ( 'NONE', #21040, 0.4606299212598425341 ) ;
#5706=CARTESIAN_POINT ( 'NONE',  ( -0.7165354330708662012, 8.847349907225958695E-17, 0.3543307086614173040 ) ) ;
#5710=ORIENTED_EDGE ( 'NONE', *, *, #17648, .F. ) ;
#5718=CARTESIAN_POINT ( 'NONE',  ( -0.2122766679520082800, -0.5838685267775929333, 0.2574827755769819038 ) ) ;
#5722=TOROIDAL_SURFACE ( 'NONE', #9773, 0.5610236220472440971, 0.1003937007874015908 ) ;
#5737=DIRECTION ( 'NONE',  ( 0.000000000000000000, 1.000000000000000000, 0.000000000000000000 ) ) ;
#5751=DIRECTION ( 'NONE',  ( 0.000000000000000000, -1.000000000000000000, 0.000000000000000000 ) ) ;
#5763=CARTESIAN_POINT ( 'NONE',  ( 0.5376957092749897749, -0.3112026930391976753, 0.2574803149606298969 ) ) ;
#5771=CARTESIAN_POINT ( 'NONE',  ( 0.4055118110236220486, 0.000000000000000000, -1.639108858267716421E-17 ) ) ;
#5787=ORIENTED_EDGE ( 'NONE', *, *, #7947, .F. ) ;
#5789=ORIENTED_EDGE ( 'NONE', *, *, #6150, .F. ) ;
#5797=CIRCLE ( 'NONE', #4862, 0.5007874015748031704 ) ;
#5816=VERTEX_POINT ( 'NONE', #6637 ) ;
#5819=AXIS2_PLACEMENT_3D ( 'NONE', #6562, #19553, #4443 ) ;
#5822=CARTESIAN_POINT ( 'NONE',  ( 0.000000000000000000, 0.000000000000000000, 0.2574803149606298969 ) ) ;
#5831=B_SPLINE_CURVE_WITH_KNOTS ( 'NONE', 3,
 ( #22998, #3617, #18303, #3192, #24817, #14090 ),
 .UNSPECIFIED., .F., .F.,
 ( 4, 2, 4 ),
 ( 0.3108507187342960387, 0.3125269569790670166, 0.3142031952238389936 ),
 .UNSPECIFIED. ) ;
#5840=CIRCLE ( 'NONE', #4908, 0.5007874015748031704 ) ;
#5854=EDGE_CURVE ( 'NONE', #27249, #24718, #5883, .T. ) ;
#5872=ORIENTED_EDGE ( 'NONE', *, *, #25236, .T. ) ;
#5877=ORIENTED_EDGE ( 'NONE', *, *, #25456, .F. ) ;
#5883=B_SPLINE_CURVE_WITH_KNOTS ( 'NONE', 3,
 ( #7270, #19990, #9234, #15889 ),
 .UNSPECIFIED., .F., .F.,
 ( 4, 4 ),
 ( 0.9359046326925629655, 0.9375808709372031036 ),
 .UNSPECIFIED. ) ;
#5896=DIRECTION ( 'NONE',  ( 0.000000000000000000, -1.000000000000000000, 0.000000000000000000 ) ) ;
#5903=CARTESIAN_POINT ( 'NONE',  ( 0.000000000000000000, 0.000000000000000000, 0.1771653543307086520 ) ) ;
#5906=FACE_BOUND ( 'NONE', #26325, .T. ) ;
#5913=VERTEX_POINT ( 'NONE', #4699 ) ;
#5918=CARTESIAN_POINT ( 'NONE',  ( -0.4143937130580483963, 0.4928070724588058393, 0.1183902030367787600 ) ) ;
#5919=PLANE ( 'NONE',  #564 ) ;
#5932=CARTESIAN_POINT ( 'NONE',  ( -0.2956505864974143805, 0.3532288989643738719, 0.1771653543307089018 ) ) ;
#5941=CIRCLE ( 'NONE', #27593, 0.5007874015748031704 ) ;
#5963=DIRECTION ( 'NONE',  ( 1.000000000000000000, 0.000000000000000000, 0.000000000000000000 ) ) ;
#5983=AXIS2_PLACEMENT_3D ( 'NONE', #4328, #17184, #19155 ) ;
#5996=CARTESIAN_POINT ( 'NONE',  ( -0.3992017438595018564, -0.2298214351608254269, 0.1771653543307087630 ) ) ;
#5999=ORIENTED_EDGE ( 'NONE', *, *, #22197, .F. ) ;
#6009=VERTEX_POINT ( 'NONE', #6970 ) ;
#6019=CARTESIAN_POINT ( 'NONE',  ( -0.0005696707463070112927, 0.4606295689977898400, 0.1771653543307085965 ) ) ;
#6020=ORIENTED_EDGE ( 'NONE', *, *, #3593, .F. ) ;
#6029=AXIS2_PLACEMENT_3D ( 'NONE', #1545, #8191, #14421 ) ;
#6038=B_SPLINE_CURVE_WITH_KNOTS ( 'NONE', 3,
 ( #13411, #5068, #7068, #323, #9437, #22173 ),
 .UNSPECIFIED., .F., .F.,
 ( 4, 2, 4 ),
 ( 0.5000000000000000000, 0.7500000000000000000, 1.000000000000000000 ),
 .UNSPECIFIED. ) ;
#6045=CARTESIAN_POINT ( 'NONE',  ( 0.0006812437162529252389, 0.6577569867597423681, 0.1461456498334882947 ) ) ;
#6066=VERTEX_POINT ( 'NONE', #2833 ) ;
#6068=CARTESIAN_POINT ( 'NONE',  ( 0.000000000000000000, 0.6212598425196850238, 0.04842519685039370358 ) ) ;
#6078=VERTEX_POINT ( 'NONE', #98 ) ;
#6083=CARTESIAN_POINT ( 'NONE',  ( 0.000000000000000000, 0.000000000000000000, 0.2574803149606298969 ) ) ;
#6090=EDGE_CURVE ( 'NONE', #17891, #18606, #13617, .T. ) ;
#6092=CARTESIAN_POINT ( 'NONE',  ( -0.5525004126151165096, 0.09742072959660473541, 0.1771653543307086520 ) ) ;
#6102=DIRECTION ( 'NONE',  ( 0.000000000000000000, 1.000000000000000000, 0.000000000000000000 ) ) ;
#6112=EDGE_CURVE ( 'NONE', #26553, #20265, #14894, .T. ) ;
#6124=VERTEX_POINT ( 'NONE', #2403 ) ;
#6133=CARTESIAN_POINT ( 'NONE',  ( 0.000000000000000000, 0.000000000000000000, 0.2574803149606298969 ) ) ;
#6150=EDGE_CURVE ( 'NONE', #18606, #14935, #5840, .T. ) ;
#6173=ORIENTED_EDGE ( 'NONE', *, *, #10087, .T. ) ;
#6189=DIRECTION ( 'NONE',  ( 0.000000000000000000, 1.000000000000000000, 0.000000000000000000 ) ) ;
#6220=CARTESIAN_POINT ( 'NONE',  ( 0.000000000000000000, 0.000000000000000000, 0.09685039370078740717 ) ) ;
#6223=SPHERICAL_SURFACE ( 'NONE', #16451, 0.1003956692913385851 ) ;
#6226=ORIENTED_EDGE ( 'NONE', *, *, #27695, .T. ) ;
#6228=CIRCLE ( 'NONE', #22006, 0.5007874015748031704 ) ;
#6234=CARTESIAN_POINT ( 'NONE',  ( 0.000000000000000000, 0.000000000000000000, 0.1771653543307086520 ) ) ;
#6240=DIRECTION ( 'NONE',  ( 1.000000000000000000, 0.000000000000000000, 0.000000000000000000 ) ) ;
#6241=ORIENTED_EDGE ( 'NONE', *, *, #3506, .T. ) ;
#6242=CARTESIAN_POINT ( 'NONE',  ( 0.000000000000000000, 0.3937007874015748254, 0.1771653543307086520 ) ) ;
#6245=AXIS2_PLACEMENT_3D ( 'NONE', #10468, #16983, #23494 ) ;
#6246=VERTEX_POINT ( 'NONE', #7733 ) ;
#6260=AXIS2_PLACEMENT_3D ( 'NONE', #19894, #22427, #15532 ) ;
#6271=FACE_OUTER_BOUND ( 'NONE', #4087, .T. ) ;
#6275=FACE_OUTER_BOUND ( 'NONE', #10466, .T. ) ;
#6310=DIRECTION ( 'NONE',  ( 0.7660444431189777914, -0.6427876096865396960, 0.000000000000000000 ) ) ;
#6312=FACE_OUTER_BOUND ( 'NONE', #15378, .T. ) ;
#6314=CARTESIAN_POINT ( 'NONE',  ( 0.0003954787107570765094, 0.5007872847596378518, 0.2574819596263889787 ) ) ;
#6320=DIRECTION ( 'NONE',  ( 0.000000000000000000, 1.000000000000000000, 0.000000000000000000 ) ) ;
#6333=CARTESIAN_POINT ( 'NONE',  ( -0.3131893444219968625, 0.3723335979320288591, 0.2467937632980442275 ) ) ;
#6352=AXIS2_PLACEMENT_3D ( 'NONE', #16420, #18080, #5549 ) ;
#6366=DIRECTION ( 'NONE',  ( 0.000000000000000000, 0.000000000000000000, 1.000000000000000000 ) ) ;
#6367=CARTESIAN_POINT ( 'NONE',  ( 0.2956505864974371400, 0.3532288989643546651, 0.1771653543307085410 ) ) ;
#6376=CARTESIAN_POINT ( 'NONE',  ( 0.3606190329934327310, 0.4297690281277732338, 0.1771653543307086520 ) ) ;
#6382=CARTESIAN_POINT ( 'NONE',  ( 0.6119360453657027854, 0.1072290460172409393, 0.2574803149606298969 ) ) ;
#6387=CIRCLE ( 'NONE', #9497, 0.01181102362204730985 ) ;
#6406=CYLINDRICAL_SURFACE ( 'NONE', #16033, 0.3937007874015748254 ) ;
#6411=CARTESIAN_POINT ( 'NONE',  ( -0.3996755081322724834, 0.4756294029998802686, 0.2574819594177531479 ) ) ;
#6413=EDGE_CURVE ( 'NONE', #11904, #12816, #22540, .T. ) ;
#6420=CIRCLE ( 'NONE', #24435, 0.4606299212598425341 ) ;
#6445=DIRECTION ( 'NONE',  ( 0.000000000000000000, -1.000000000000000000, 0.000000000000000000 ) ) ;
#6451=VERTEX_POINT ( 'NONE', #14673 ) ;
#6456=CARTESIAN_POINT ( 'NONE',  ( 0.4563437505067101663, 0.07988585396536060368, 0.1494804571663867210 ) ) ;
#6459=EDGE_CURVE ( 'NONE', #478, #14228, #5146, .T. ) ;
#6464=CARTESIAN_POINT ( 'NONE',  ( -0.6339803004441102452, 0.1124719464476266473, 0.1183902030382474879 ) ) ;
#6477=VERTEX_POINT ( 'NONE', #24358 ) ;
#6483=CARTESIAN_POINT ( 'NONE',  ( 0.4126915023378835423, -0.2375990494930988739, 0.2330651857771384172 ) ) ;
#6489=AXIS2_PLACEMENT_3D ( 'NONE', #15563, #6520, #15152 ) ;
#6490=CARTESIAN_POINT ( 'NONE',  ( 0.0004405150045524555734, 0.6212597256746514862, 0.2574819594177531479 ) ) ;
#6495=CARTESIAN_POINT ( 'NONE',  ( 0.3214446924536846772, 0.3840069416942866742, 0.09685039370078740717 ) ) ;
#6502=EDGE_LOOP ( 'NONE', ( #1870, #22867 ) ) ;
#6504=FACE_OUTER_BOUND ( 'NONE', #5555, .T. ) ;
#6513=CARTESIAN_POINT ( 'NONE',  ( 0.3122922550372661532, 0.3730863453251304085, 0.2467937633102478545 ) ) ;
#6520=DIRECTION ( 'NONE',  ( 0.000000000000000000, 0.000000000000000000, -1.000000000000000000 ) ) ;
#6529=CARTESIAN_POINT ( 'NONE',  ( 0.6117062799105453808, 0.1085321106658576895, 0.09685039370078740717 ) ) ;
#6540=B_SPLINE_CURVE_WITH_KNOTS ( 'NONE', 3,
 ( #22455, #17908, #7342, #3082, #22040, #11715, #26977, #26830, #7480, #7628 ),
 .UNSPECIFIED., .F., .F.,
 ( 4, 2, 2, 2, 4 ),
 ( 0.000000000000000000, 0.2500000000000000000, 0.5000000000000000000, 0.7500000000000000000, 1.000000000000000000 ),
 .UNSPECIFIED. ) ;
#6541=DIRECTION ( 'NONE',  ( 1.000000000000000000, 0.000000000000000000, 0.000000000000000000 ) ) ;
#6543=AXIS2_PLACEMENT_3D ( 'NONE', #27100, #14253, #16635 ) ;
#6546=AXIS2_PLACEMENT_3D ( 'NONE', #25374, #1781, #23557 ) ;
#6547=CARTESIAN_POINT ( 'NONE',  ( -0.6119360453657125554, 0.1072290460171901605, 0.09685039370078740717 ) ) ;
#6550=CARTESIAN_POINT ( 'NONE',  ( -0.4339912984563299436, -0.2498791196563492356, 0.2574803149606298969 ) ) ;
#6562=CARTESIAN_POINT ( 'NONE',  ( 0.3606190329934327310, 0.4297690281277732338, 0.1771653543307086520 ) ) ;
#6571=CARTESIAN_POINT ( 'NONE',  ( 0.2131049448083992270, -0.5835666837866889667, 0.09685039370078740717 ) ) ;
#6574=VERTEX_POINT ( 'NONE', #8967 ) ;
#6578=CARTESIAN_POINT ( 'NONE',  ( -0.4126915023499354573, -0.2375990495000580294, 0.1212655228631613069 ) ) ;
#6579=ADVANCED_FACE ( 'NONE', ( #9227 ), #2684, .F. ) ;
#6586=EDGE_CURVE ( 'NONE', #833, #15551, #2119, .T. ) ;
#6590=CARTESIAN_POINT ( 'NONE',  ( 0.5610236220472440971, 0.000000000000000000, 0.1771653543307086520 ) ) ;
#6592=CARTESIAN_POINT ( 'NONE',  ( -0.6117062799105531523, 0.1085321106658068829, 0.2574803149606298969 ) ) ;
#6595=DIRECTION ( 'NONE',  ( 1.000000000000000000, 0.000000000000000000, 0.000000000000000000 ) ) ;
#6596=VERTEX_POINT ( 'NONE', #25101 ) ;
#6602=CARTESIAN_POINT ( 'NONE',  ( 0.000000000000000000, 0.000000000000000000, 0.1771653543307086520 ) ) ;
#6615=EDGE_CURVE ( 'NONE', #11455, #6009, #5831, .T. ) ;
#6634=EDGE_CURVE ( 'NONE', #24688, #2747, #2234, .T. ) ;
#6637=CARTESIAN_POINT ( 'NONE',  ( -4.821444091131312140E-17, -0.3937007874015748254, 0.01181102362204724393 ) ) ;
#6640=EDGE_LOOP ( 'NONE', ( #442, #16200 ) ) ;
#6644=CARTESIAN_POINT ( 'NONE',  ( 0.000000000000000000, 0.000000000000000000, -3.278217716535432842E-17 ) ) ;
#6651=ORIENTED_EDGE ( 'NONE', *, *, #3902, .F. ) ;
#6679=VERTEX_POINT ( 'NONE', #26416 ) ;
#6685=CARTESIAN_POINT ( 'NONE',  ( -0.6117062799105453808, 0.1085321106658580781, 0.09685039370078740717 ) ) ;
#6707=ORIENTED_EDGE ( 'NONE', *, *, #23893, .F. ) ;
#6711=VERTEX_POINT ( 'NONE', #5356 ) ;
#6713=ORIENTED_EDGE ( 'NONE', *, *, #22297, .F. ) ;
#6719=DIRECTION ( 'NONE',  ( 0.000000000000000000, 0.000000000000000000, 1.000000000000000000 ) ) ;
#6732=EDGE_CURVE ( 'NONE', #19560, #18356, #760, .T. ) ;
#6740=DIMENSIONAL_EXPONENTS ( 1.000000000000000000, 0.000000000000000000, 0.000000000000000000, 0.000000000000000000, 0.000000000000000000, 0.000000000000000000, 0.000000000000000000 ) ;
#6769=CARTESIAN_POINT ( 'NONE',  ( -0.2128972891168661452, -0.5836425148029424914, 0.09684874924366436433 ) ) ;
#6776=DIRECTION ( 'NONE',  ( -0.3420201433256691570, -0.9396926207859082059, 0.000000000000000000 ) ) ;
#6783=CARTESIAN_POINT ( 'NONE',  ( -0.1580799066051627177, -0.4326553680327468454, 0.1771653543307088186 ) ) ;
#6802=EDGE_CURVE ( 'NONE', #4649, #8161, #25738, .T. ) ;
#6819=ORIENTED_EDGE ( 'NONE', *, *, #2646, .F. ) ;
#6820=CARTESIAN_POINT ( 'NONE',  ( 0.000000000000000000, 0.000000000000000000, 0.2574803149606298969 ) ) ;
#6832=ORIENTED_EDGE ( 'NONE', *, *, #3694, .T. ) ;
#6834=LINE ( 'NONE', #24456, #23658 ) ;
#6848=CARTESIAN_POINT ( 'NONE',  ( 0.3991696156513425686, 0.4760540497244023506, 0.2574827755769819038 ) ) ;
#6854=ORIENTED_EDGE ( 'NONE', *, *, #3309, .T. ) ;
#6863=DIRECTION ( 'NONE',  ( 1.000000000000000000, 0.000000000000000000, 0.000000000000000000 ) ) ;
#6881=ORIENTED_EDGE ( 'NONE', *, *, #4467, .F. ) ;
#6893=FACE_OUTER_BOUND ( 'NONE', #12536, .T. ) ;
#6903=CARTESIAN_POINT ( 'NONE',  ( 0.000000000000000000, 0.000000000000000000, 0.09685039370078740717 ) ) ;
#6928=ORIENTED_EDGE ( 'NONE', *, *, #23042, .F. ) ;
#6934=DIRECTION ( 'NONE',  ( 0.000000000000000000, 0.000000000000000000, 1.000000000000000000 ) ) ;
#6935=CIRCLE ( 'NONE', #6029, 0.5007874015748031704 ) ;
#6947=DIRECTION ( 'NONE',  ( 0.000000000000000000, 0.000000000000000000, 1.000000000000000000 ) ) ;
#6954=CARTESIAN_POINT ( 'NONE',  ( 0.000000000000000000, 0.000000000000000000, 0.09685039370078740717 ) ) ;
#6958=AXIS2_PLACEMENT_3D ( 'NONE', #16284, #20938, #25166 ) ;
#6960=ORIENTED_EDGE ( 'NONE', *, *, #25396, .T. ) ;
#6962=CARTESIAN_POINT ( 'NONE',  ( -0.6118597084614606496, 0.1076640027107484132, 0.09684793308443542803 ) ) ;
#6967=B_SPLINE_CURVE_WITH_KNOTS ( 'NONE', 3,
 ( #20360, #9324, #26562, #16131, #7219, #15838 ),
 .UNSPECIFIED., .F., .F.,
 ( 4, 2, 4 ),
 ( 0.9031406754215589583, 0.9046454396443730506, 0.9061502038671860326 ),
 .UNSPECIFIED. ) ;
#6970=CARTESIAN_POINT ( 'NONE',  ( -0.5376957092749645728, -0.3112026930392425284, 0.09685039370078740717 ) ) ;
#6981=CARTESIAN_POINT ( 'NONE',  ( 0.000000000000000000, 0.000000000000000000, 0.3425196850393700809 ) ) ;
#6989=CARTESIAN_POINT ( 'NONE',  ( 0.3996755081323252745, 0.4756294029998354156, 0.2574819594177527593 ) ) ;
#6996=EDGE_CURVE ( 'NONE', #14064, #16332, #13083, .T. ) ;
#7003=ORIENTED_EDGE ( 'NONE', *, *, #4708, .F. ) ;
#7006=AXIS2_PLACEMENT_3D ( 'NONE', #19227, #2401, #25449 ) ;
#7033=ORIENTED_EDGE ( 'NONE', *, *, #746, .T. ) ;
#7037=CARTESIAN_POINT ( 'NONE',  ( -0.2126900928101059240, -0.5837180524351401889, 0.09684793308443542803 ) ) ;
#7044=AXIS2_PLACEMENT_3D ( 'NONE', #7244, #5418, #15863 ) ;
#7051=CARTESIAN_POINT ( 'NONE',  ( -0.4932821129636645874, 0.08637579872942342807, 0.2574803149606298969 ) ) ;
#7052=ORIENTED_EDGE ( 'NONE', *, *, #15524, .F. ) ;
#7068=CARTESIAN_POINT ( 'NONE',  ( -0.4015002836674314013, -0.2311469024290320751, 0.2048502514845859379 ) ) ;
#7070=CARTESIAN_POINT ( 'NONE',  ( -6.132876883919029269E-17, -0.5007874015748031704, -3.278217716535432842E-17 ) ) ;
#7092=FACE_OUTER_BOUND ( 'NONE', #437, .T. ) ;
#7093=ORIENTED_EDGE ( 'NONE', *, *, #3867, .F. ) ;
#7104=B_SPLINE_CURVE_WITH_KNOTS ( 'NONE', 3,
 ( #15325, #6411, #15038, #4289, #26034, #23654 ),
 .UNSPECIFIED., .F., .F.,
 ( 4, 2, 4 ),
 ( 0.9359046326925629655, 0.9375808709372039917, 0.9392571091818440188 ),
 .UNSPECIFIED. ) ;
#7107=CARTESIAN_POINT ( 'NONE',  ( -0.4561454261039838420, 0.08101060747556922126, 0.2048502514525085139 ) ) ;
#7110=CARTESIAN_POINT ( 'NONE',  ( 0.1718374205099799101, -0.4703827404237102550, 0.2574803149606298969 ) ) ;
#7113=CARTESIAN_POINT ( 'NONE',  ( -0.0006832381873097717172, 0.6614169699448725348, 0.1926811207749853927 ) ) ;
#7115=DIRECTION ( 'NONE',  ( 0.3420201433256690460, -0.9396926207859084279, 0.000000000000000000 ) ) ;
#7123=CARTESIAN_POINT ( 'NONE',  ( -0.1918813796216842782, -0.5271897577243779276, 0.1771653543307086520 ) ) ;
#7124=DIRECTION ( 'NONE',  ( -0.5000000000000001110, 0.8660254037844384856, 0.000000000000000000 ) ) ;
#7125=CARTESIAN_POINT ( 'NONE',  ( 0.0005696707463077370576, 0.4606295689977898400, 0.1771653543307089018 ) ) ;
#7149=DIRECTION ( 'NONE',  ( 0.000000000000000000, 0.000000000000000000, 1.000000000000000000 ) ) ;
#7181=EDGE_LOOP ( 'NONE', ( #18090, #23493 ) ) ;
#7200=EDGE_CURVE ( 'NONE', #478, #3160, #17594, .T. ) ;
#7207=DIRECTION ( 'NONE',  ( 1.000000000000000000, 0.000000000000000000, 0.000000000000000000 ) ) ;
#7211=EDGE_LOOP ( 'NONE', ( #85, #24786 ) ) ;
#7217=CARTESIAN_POINT ( 'NONE',  ( 0.000000000000000000, 0.000000000000000000, 0.01181102362204724393 ) ) ;
#7219=CARTESIAN_POINT ( 'NONE',  ( 0.4338922498494567348, -0.2500511477696476526, 0.2574819596263889787 ) ) ;
#7222=ADVANCED_FACE ( 'NONE', ( #18294 ), #23038, .F. ) ;
#7231=AXIS2_PLACEMENT_3D ( 'NONE', #24459, #5112, #13736 ) ;
#7244=CARTESIAN_POINT ( 'NONE',  ( 0.5525004126151165096, 0.09742072959660433296, 0.1771653543307086520 ) ) ;
#7253=CARTESIAN_POINT ( 'NONE',  ( 0.5579526598176609564, -0.3213561723288210215, 0.1183902030407611161 ) ) ;
#7263=ADVANCED_FACE ( 'NONE', ( #5319 ), #9949, .F. ) ;
#7270=CARTESIAN_POINT ( 'NONE',  ( -0.0006615832605804723319, 0.6212594902576319411, 0.2574803149606298969 ) ) ;
#7277=CARTESIAN_POINT ( 'NONE',  ( 0.3998447049182496382, 0.4754871227240771714, 0.09685039370078740717 ) ) ;
#7281=CARTESIAN_POINT ( 'NONE',  ( 0.000000000000000000, 0.000000000000000000, 0.09685039370078740717 ) ) ;
#7282=VERTEX_POINT ( 'NONE', #19743 ) ;
#7291=CARTESIAN_POINT ( 'NONE',  ( 0.000000000000000000, 0.5007874015748031704, -3.278217716535432842E-17 ) ) ;
#7300=EDGE_CURVE ( 'NONE', #6574, #11007, #20770, .T. ) ;
#7301=CARTESIAN_POINT ( 'NONE',  ( 0.3606190329934327310, 0.4297690281277732338, 0.07676968503937006694 ) ) ;
#7302=CARTESIAN_POINT ( 'NONE',  ( 0.3998447049182889956, 0.4754871227240441423, 0.2574803149606298969 ) ) ;
#7310=CARTESIAN_POINT ( 'NONE',  ( -0.3988311005573134116, 0.4763376377694984454, 0.09685039370078740717 ) ) ;
#7317=CARTESIAN_POINT ( 'NONE',  ( 0.3986320731132085293, -0.2308081338369910029, 0.1639447408811634532 ) ) ;
#7328=ORIENTED_EDGE ( 'NONE', *, *, #13134, .F. ) ;
#7342=CARTESIAN_POINT ( 'NONE',  ( -0.4133615125900214071, 0.4936731914959181511, 0.2359405056196126338 ) ) ;
#7345=CYLINDRICAL_SURFACE ( 'NONE', #17731, 0.6212598425196850238 ) ;
#7353=CARTESIAN_POINT ( 'NONE',  ( 0.6119360453657125554, 0.1072290460171897442, 0.09685039370078740717 ) ) ;
#7371=ORIENTED_EDGE ( 'NONE', *, *, #3867, .T. ) ;
#7378=DIRECTION ( 'NONE',  ( 0.000000000000000000, -1.000000000000000000, 0.000000000000000000 ) ) ;
#7383=CARTESIAN_POINT ( 'NONE',  ( 0.1669561253493014596, -0.4569961989609055975, 0.2467937633349458482 ) ) ;
#7385=ORIENTED_EDGE ( 'NONE', *, *, #8608, .F. ) ;
#7423=VERTEX_POINT ( 'NONE', #20011 ) ;
#7430=ORIENTED_EDGE ( 'NONE', *, *, #26186, .T. ) ;
#7433=CIRCLE ( 'NONE', #5674, 0.5007874015748031704 ) ;
#7446=ADVANCED_FACE ( 'NONE', ( #6893, #18001 ), #20432, .T. ) ;
#7463=B_SPLINE_CURVE_WITH_KNOTS ( 'NONE', 3,
 ( #15816, #26530, #26677, #9436 ),
 .UNSPECIFIED., .F., .F.,
 ( 4, 4 ),
 ( 0.3125269569790670721, 0.3142031952238389936 ),
 .UNSPECIFIED. ) ;
#7480=CARTESIAN_POINT ( 'NONE',  ( -0.4068047116056149881, 0.4858504993699251928, 0.1061598535658933862 ) ) ;
#7490=CARTESIAN_POINT ( 'NONE',  ( -0.2131049448084480213, -0.5835666837866708700, 0.2574803149606298969 ) ) ;
#7513=DIRECTION ( 'NONE',  ( 0.000000000000000000, 0.000000000000000000, 1.000000000000000000 ) ) ;
#7520=FACE_OUTER_BOUND ( 'NONE', #221, .T. ) ;
#7526=FACE_BOUND ( 'NONE', #21577, .T. ) ;
#7528=DIRECTION ( 'NONE',  ( -0.5000000000000002220, -0.8660254037844384856, 0.000000000000000000 ) ) ;
#7551=EDGE_CURVE ( 'NONE', #6711, #17345, #15394, .T. ) ;
#7576=AXIS2_PLACEMENT_3D ( 'NONE', #25558, #8329, #10284 ) ;
#7596=FACE_OUTER_BOUND ( 'NONE', #17849, .T. ) ;
#7599=B_SPLINE_CURVE_WITH_KNOTS ( 'NONE', 3,
 ( #7277, #12079, #19130, #20833, #12219, #27482 ),
 .UNSPECIFIED., .F., .F.,
 ( 4, 2, 4 ),
 ( 0.3108507187342950395, 0.3125269569790680158, 0.3142031952238389936 ),
 .UNSPECIFIED. ) ;
#7606=VECTOR ( 'NONE', #2138, 39.37007874015748143 ) ;
#7614=EDGE_LOOP ( 'NONE', ( #18759, #18029 ) ) ;
#7617=CARTESIAN_POINT ( 'NONE',  ( 0.4334967711386992772, -0.2507361369899905879, 0.09684874903502814492 ) ) ;
#7626=AXIS2_PLACEMENT_3D ( 'NONE', #8424, #17044, #21423 ) ;
#7627=EDGE_CURVE ( 'NONE', #6066, #24915, #19437, .T. ) ;
#7628=CARTESIAN_POINT ( 'NONE',  ( -0.3988311005573134116, 0.4763376377694984454, 0.09685039370078740717 ) ) ;
#7631=ADVANCED_FACE ( 'NONE', ( #9971, #18571 ), #20715, .T. ) ;
#7649=B_SPLINE_CURVE_WITH_KNOTS ( 'NONE', 3,
 ( #15484, #13342, #21968, #22100, #26463, #7125 ),
 .UNSPECIFIED., .F., .F.,
 ( 4, 2, 4 ),
 ( 0.000000000000000000, 0.2500000000000000000, 0.5000000000000000000 ),
 .UNSPECIFIED. ) ;
#7666=DIRECTION ( 'NONE',  ( 0.000000000000000000, 1.000000000000000000, 0.000000000000000000 ) ) ;
#7692=FACE_OUTER_BOUND ( 'NONE', #14145, .T. ) ;
#7701=EDGE_CURVE ( 'NONE', #23891, #18882, #3182, .T. ) ;
#7708=ORIENTED_EDGE ( 'NONE', *, *, #1280, .T. ) ;
#7731=CARTESIAN_POINT ( 'NONE',  ( 0.3223547283257516272, 0.3832433309296771617, 0.2574803149606298969 ) ) ;
#7733=CARTESIAN_POINT ( 'NONE',  ( -0.3988311005573527690, 0.4763376377694653607, 0.2574803149606298969 ) ) ;
#7737=CARTESIAN_POINT ( 'NONE',  ( 0.4790450267203003598, 0.08506312950115990645, 0.1075369453498891542 ) ) ;
#7740=CARTESIAN_POINT ( 'NONE',  ( -0.5379168165870180651, -0.3108204284649448423, 0.2574827755769819038 ) ) ;
#7741=CARTESIAN_POINT ( 'NONE',  ( -0.4790450267015415875, 0.08506312949784111677, 0.1075369453641766698 ) ) ;
#7753=CARTESIAN_POINT ( 'NONE',  ( 0.2243259791912049217, -0.6183223858000764794, 0.1461456498277223237 ) ) ;
#7755=DIRECTION ( 'NONE',  ( 0.000000000000000000, -1.000000000000000000, 0.000000000000000000 ) ) ;
#7760=CARTESIAN_POINT ( 'NONE',  ( 0.4339912984563291110, -0.2498791196563492356, 0.09685039370078740717 ) ) ;
#7773=ORIENTED_EDGE ( 'NONE', *, *, #9099, .F. ) ;
#7782=CARTESIAN_POINT ( 'NONE',  ( 0.2956505864974370290, 0.3532288989643546095, 0.1639447408648230242 ) ) ;
#7788=EDGE_LOOP ( 'NONE', ( #1013, #7093, #10922, #23915, #20878, #941 ) ) ;
#7793=CARTESIAN_POINT ( 'NONE',  ( -0.2255758929756846998, -0.6217623271424783660, 0.1926811207753210409 ) ) ;
#7810=DIRECTION ( 'NONE',  ( 0.000000000000000000, 0.000000000000000000, -1.000000000000000000 ) ) ;
#7811=AXIS2_PLACEMENT_3D ( 'NONE', #24026, #20060, #4944 ) ;
#7844=ORIENTED_EDGE ( 'NONE', *, *, #27521, .T. ) ;
#7875=CARTESIAN_POINT ( 'NONE',  ( 0.4688657571939683910, 0.08326155277437964630, 0.1212655228563162269 ) ) ;
#7877=CARTESIAN_POINT ( 'NONE',  ( -0.2965233727166468047, 0.3524965443697193335, 0.1771653543307085965 ) ) ;
#7886=TOROIDAL_SURFACE ( 'NONE', #20941, 0.5610236220472440971, 0.1003937007874015908 ) ;
#7892=CARTESIAN_POINT ( 'NONE',  ( 0.2161007281681049663, -0.5956855348339761269, 0.2481708550939305813 ) ) ;
#7905=B_SPLINE_CURVE_WITH_KNOTS ( 'NONE', 3,
 ( #832, #7892, #9561, #973, #24829, #1253, #7753, #14260, #22290, #16366 ),
 .UNSPECIFIED., .F., .F.,
 ( 4, 2, 2, 2, 4 ),
 ( 0.000000000000000000, 0.2500000000000003331, 0.5000000000000002220, 0.7500000000000001110, 1.000000000000000000 ),
 .UNSPECIFIED. ) ;
#7910=CARTESIAN_POINT ( 'NONE',  ( 0.000000000000000000, 0.000000000000000000, 0.01181102362204724393 ) ) ;
#7917=AXIS2_PLACEMENT_3D ( 'NONE', #9035, #15818, #15286 ) ;
#7923=DIRECTION ( 'NONE',  ( 1.000000000000000000, 0.000000000000000000, 0.000000000000000000 ) ) ;
#7935=CARTESIAN_POINT ( 'NONE',  ( 0.4932821129636645874, 0.08637579872942321990, 0.2574803149606298969 ) ) ;
#7947=EDGE_CURVE ( 'NONE', #9216, #15905, #7649, .T. ) ;
#7965=ORIENTED_EDGE ( 'NONE', *, *, #16918, .T. ) ;
#7969=DIRECTION ( 'NONE',  ( 0.000000000000000000, 1.000000000000000000, 0.000000000000000000 ) ) ;
#7977=TOROIDAL_SURFACE ( 'NONE', #23775, 0.5610236220472440971, 0.1003937007874015908 ) ;
#7979=DIMENSIONAL_EXPONENTS ( 1.000000000000000000, 0.000000000000000000, 0.000000000000000000, 0.000000000000000000, 0.000000000000000000, 0.000000000000000000, 0.000000000000000000 ) ;
#7982=EDGE_CURVE ( 'NONE', #6078, #2920, #25303, .T. ) ;
#7992=( NAMED_UNIT ( * ) PLANE_ANGLE_UNIT ( ) SI_UNIT ( $, .RADIAN. ) ) ;
#8013=SPHERICAL_SURFACE ( 'NONE', #9328, 0.1003956692913385851 ) ;
#8031=CARTESIAN_POINT ( 'NONE',  ( 0.5610236220472440971, 0.000000000000000000, 0.1771653543307086520 ) ) ;
#8034=ORIENTED_EDGE ( 'NONE', *, *, #26906, .T. ) ;
#8042=EDGE_CURVE ( 'NONE', #5560, #20533, #14985, .T. ) ;
#8048=EDGE_LOOP ( 'NONE', ( #26457, #8589, #22907, #24505, #23074 ) ) ;
#8052=CARTESIAN_POINT ( 'NONE',  ( 0.0005939837304750000086, 0.5007870493127504208, 0.09685039370078740717 ) ) ;
#8064=CIRCLE ( 'NONE', #2121, 0.6212598425196850238 ) ;
#8070=VERTEX_POINT ( 'NONE', #5570 ) ;
#8071=DIRECTION ( 'NONE',  ( 1.000000000000000000, 0.000000000000000000, 0.000000000000000000 ) ) ;
#8075=ORIENTED_EDGE ( 'NONE', *, *, #17839, .F. ) ;
#8078=AXIS2_PLACEMENT_3D ( 'NONE', #16218, #1110, #5479 ) ;
#8079=TOROIDAL_SURFACE ( 'NONE', #2651, 0.5610236220472440971, 0.1003937007874015908 ) ;
#8083=CARTESIAN_POINT ( 'NONE',  ( -0.1623262587461356543, -0.4476804331100887602, 0.1212655228106225697 ) ) ;
#8098=VERTEX_POINT ( 'NONE', #27751 ) ;
#8108=DIRECTION ( 'NONE',  ( 0.000000000000000000, 0.000000000000000000, 1.000000000000000000 ) ) ;
#8128=DIRECTION ( 'NONE',  ( 0.000000000000000000, 1.000000000000000000, 0.000000000000000000 ) ) ;
#8129=AXIS2_PLACEMENT_3D ( 'NONE', #20253, #3284, #27044 ) ;
#8130=ORIENTED_EDGE ( 'NONE', *, *, #24794, .T. ) ;
#8141=ADVANCED_FACE ( 'NONE', ( #6275 ), #18972, .T. ) ;
#8149=DIRECTION ( 'NONE',  ( 0.000000000000000000, 0.000000000000000000, -1.000000000000000000 ) ) ;
#8161=VERTEX_POINT ( 'NONE', #26269 ) ;
#8165=DIRECTION ( 'NONE',  ( 1.000000000000000000, 0.000000000000000000, 0.000000000000000000 ) ) ;
#8185=CARTESIAN_POINT ( 'NONE',  ( -0.0005696707463070112927, 0.4606295689977898400, 0.1771653543307085965 ) ) ;
#8191=DIRECTION ( 'NONE',  ( 0.000000000000000000, 0.000000000000000000, 1.000000000000000000 ) ) ;
#8211=EDGE_CURVE ( 'NONE', #24915, #5352, #12624, .T. ) ;
#8222=CARTESIAN_POINT ( 'NONE',  ( 0.5484420430273854175, -0.3174147232949027786, 0.2481708550944002056 ) ) ;
#8241=CARTESIAN_POINT ( 'NONE',  ( 0.000000000000000000, 0.000000000000000000, 0.01181102362204724393 ) ) ;
#8261=EDGE_LOOP ( 'NONE', ( #25645, #20342, #3086, #16725, #18542, #10519 ) ) ;
#8264=DIRECTION ( 'NONE',  ( -0.3420201433256691570, 0.9396926207859084279, 0.000000000000000000 ) ) ;
#8272=CARTESIAN_POINT ( 'NONE',  ( -0.4535326485287287657, 0.08054850140359764987, 0.1771653543307088186 ) ) ;
#8274=CARTESIAN_POINT ( 'NONE',  ( 0.4210617728748768385, -0.2437762437830508222, 0.2467937632988287666 ) ) ;
#8282=CARTESIAN_POINT ( 'NONE',  ( -0.5376957092749378164, -0.3112026930392873814, 0.2574803149606298969 ) ) ;
#8288=DIRECTION ( 'NONE',  ( 1.224646799147353207E-16, 1.000000000000000000, -0.000000000000000000 ) ) ;
#8301=CARTESIAN_POINT ( 'NONE',  ( -0.0005696707463066808278, 0.4606295689977896735, 0.1639447408835300324 ) ) ;
#8302=AXIS2_PLACEMENT_3D ( 'NONE', #16921, #25531, #10123 ) ;
#8311=VERTEX_POINT ( 'NONE', #5429 ) ;
#8314=ADVANCED_FACE ( 'NONE', ( #4855, #18397 ), #22099, .T. ) ;
#8323=ORIENTED_EDGE ( 'NONE', *, *, #7982, .T. ) ;
#8325=B_SPLINE_CURVE_WITH_KNOTS ( 'NONE', 3,
 ( #24728, #13716, #5391, #11597, #882, #7793, #27423, #3529, #1293, #25300 ),
 .UNSPECIFIED., .F., .F.,
 ( 4, 2, 2, 2, 4 ),
 ( 0.000000000000000000, 0.2499999999999997780, 0.5000000000000000000, 0.7500000000000002220, 1.000000000000000000 ),
 .UNSPECIFIED. ) ;
#8329=DIRECTION ( 'NONE',  ( 0.6427876096865391409, -0.7660444431189782355, 0.000000000000000000 ) ) ;
#8338=ADVANCED_FACE ( 'NONE', ( #7692 ), #12699, .T. ) ;
#8348=ORIENTED_EDGE ( 'NONE', *, *, #16773, .F. ) ;
#8352=DIRECTION ( 'NONE',  ( 0.000000000000000000, 0.000000000000000000, 1.000000000000000000 ) ) ;
#8354=DIRECTION ( 'NONE',  ( 1.000000000000000000, 0.000000000000000000, 0.000000000000000000 ) ) ;
#8365=DIRECTION ( 'NONE',  ( 0.000000000000000000, 1.000000000000000000, 0.000000000000000000 ) ) ;
#8381=DIRECTION ( 'NONE',  ( 0.000000000000000000, 1.000000000000000000, 0.000000000000000000 ) ) ;
#8400=AXIS2_PLACEMENT_3D ( 'NONE', #6234, #8352, #25854 ) ;
#8403=ORIENTED_EDGE ( 'NONE', *, *, #16269, .T. ) ;
#8415=CARTESIAN_POINT ( 'NONE',  ( -0.5692936381921454014, -0.3294684677441130360, 0.1461456498322906972 ) ) ;
#8424=CARTESIAN_POINT ( 'NONE',  ( 0.000000000000000000, 0.000000000000000000, 0.3425196850393700809 ) ) ;
#8429=EDGE_CURVE ( 'NONE', #13907, #5352, #5941, .T. ) ;
#8434=AXIS2_PLACEMENT_3D ( 'NONE', #18536, #1195, #27042 ) ;
#8458=CARTESIAN_POINT ( 'NONE',  ( 0.1570092758121679200, -0.4330450457732857861, 0.1771653543307087630 ) ) ;
#8459=ORIENTED_EDGE ( 'NONE', *, *, #17268, .F. ) ;
#8485=EDGE_CURVE ( 'NONE', #6596, #22691, #15881, .T. ) ;
#8489=DIRECTION ( 'NONE',  ( 0.000000000000000000, 0.000000000000000000, 1.000000000000000000 ) ) ;
#8500=CARTESIAN_POINT ( 'NONE',  ( 0.6241612306989096082, 0.1093779649447741559, 0.2481708550952254622 ) ) ;
#8501=CARTESIAN_POINT ( 'NONE',  ( -0.5376957092749378164, -0.3112026930392873814, 0.2574803149606298969 ) ) ;
#8531=PRODUCT_DEFINITION_CONTEXT ( 'detailed design', #14720, 'design' ) ;
#8537=FACE_BOUND ( 'NONE', #24114, .T. ) ;
#8555=CARTESIAN_POINT ( 'NONE',  ( -0.5484420430267122892, -0.3174147232945255803, 0.2481708550949786873 ) ) ;
#8557=ORIENTED_EDGE ( 'NONE', *, *, #10907, .F. ) ;
#8568=ORIENTED_EDGE ( 'NONE', *, *, #23619, .T. ) ;
#8569=CARTESIAN_POINT ( 'NONE',  ( -0.4790450267014849661, 0.08506312949783263744, 0.2467937632971976825 ) ) ;
#8579=CARTESIAN_POINT ( 'NONE',  ( -0.6239291699170932404, 0.1106940470470682975, 0.2481708550940099900 ) ) ;
#8589=ORIENTED_EDGE ( 'NONE', *, *, #21703, .T. ) ;
#8593=ORIENTED_EDGE ( 'NONE', *, *, #22305, .T. ) ;
#8598=CARTESIAN_POINT ( 'NONE',  ( 0.1623262587483975672, -0.4476804331163366513, 0.2330651858608774607 ) ) ;
#8601=CARTESIAN_POINT ( 'NONE',  ( -0.2131049448083992270, -0.5835666837866889667, 0.09685039370078740717 ) ) ;
#8608=EDGE_CURVE ( 'NONE', #21729, #15613, #24305, .T. ) ;
#8614=EDGE_CURVE ( 'NONE', #10869, #17871, #6420, .T. ) ;
#8618=EDGE_CURVE ( 'NONE', #12716, #6246, #7104, .T. ) ;
#8623=FACE_BOUND ( 'NONE', #14820, .T. ) ;
#8625=CARTESIAN_POINT ( 'NONE',  ( -0.4338922498494567348, -0.2500511477696472085, 0.09684874903502814492 ) ) ;
#8646=AXIS2_PLACEMENT_3D ( 'NONE', #4993, #13616, #22235 ) ;
#8654=VECTOR ( 'NONE', #3675, 39.37007874015748143 ) ;
#8658=DIRECTION ( 'NONE',  ( -0.1736481776669313026, -0.9848077530122080203, 0.000000000000000000 ) ) ;
#8660=CARTESIAN_POINT ( 'NONE',  ( 0.1707210962531913734, -0.4707890492249701131, 0.09685039370078740717 ) ) ;
#8670=ADVANCED_BREP_SHAPE_REPRESENTATION ( 'Deep Groove Ball Bearing 20x37x9', ( #22049, #11588 ), #25599 ) ;
#8673=AXIS2_PLACEMENT_3D ( 'NONE', #21001, #27087, #852 ) ;
#8691=CARTESIAN_POINT ( 'NONE',  ( -0.4216473064036311280, -0.2427620699869365573, 0.1075369453531297426 ) ) ;
#8711=EDGE_CURVE ( 'NONE', #12716, #20920, #5043, .T. ) ;
#8721=FACE_BOUND ( 'NONE', #16644, .T. ) ;
#8728=ORIENTED_EDGE ( 'NONE', *, *, #3742, .F. ) ;
#8734=DIRECTION ( 'NONE',  ( 0.000000000000000000, 1.000000000000000000, 0.000000000000000000 ) ) ;
#8740=AXIS2_PLACEMENT_3D ( 'NONE', #7910, #20761, #14274 ) ;
#8741=CARTESIAN_POINT ( 'NONE',  ( 0.0006615832605804723319, 0.6212594902576319411, 0.2574803149606298969 ) ) ;
#8763=DIRECTION ( 'NONE',  ( 0.000000000000000000, -1.000000000000000000, 0.000000000000000000 ) ) ;
#8767=CARTESIAN_POINT ( 'NONE',  ( -0.1718374205099799101, -0.4703827404237102550, 0.09685039370078740717 ) ) ;
#8787=ORIENTED_EDGE ( 'NONE', *, *, #6802, .T. ) ;
#8793=CARTESIAN_POINT ( 'NONE',  ( -0.4334967711386992772, -0.2507361369899905879, 0.2574819596263889787 ) ) ;
#8796=DIRECTION ( 'NONE',  ( 0.000000000000000000, 0.000000000000000000, 1.000000000000000000 ) ) ;
#8815=ORIENTED_EDGE ( 'NONE', *, *, #19826, .F. ) ;
#8847=EDGE_LOOP ( 'NONE', ( #11177, #19226, #26433, #1079 ) ) ;
#8857=CARTESIAN_POINT ( 'NONE',  ( 0.6117448998508543401, 0.1083144418130956715, 0.09684874924366436433 ) ) ;
#8877=DIRECTION ( 'NONE',  ( 1.000000000000000000, 0.000000000000000000, 0.000000000000000000 ) ) ;
#8888=DIRECTION ( 'NONE',  ( 1.000000000000000000, 0.000000000000000000, 0.000000000000000000 ) ) ;
#8893=ORIENTED_EDGE ( 'NONE', *, *, #7982, .F. ) ;
#8924=VERTEX_POINT ( 'NONE', #1988 ) ;
#8934=VERTEX_POINT ( 'NONE', #10748 ) ;
#8955=SPHERICAL_SURFACE ( 'NONE', #21055, 0.1003956692913385851 ) ;
#8956=CARTESIAN_POINT ( 'NONE',  ( 0.000000000000000000, 0.5007874015748031704, 0.3059055118110236560 ) ) ;
#8967=CARTESIAN_POINT ( 'NONE',  ( -7.608238775805210269E-17, -0.6212598425196850238, -3.278217716535432842E-17 ) ) ;
#8978=EDGE_CURVE ( 'NONE', #14228, #4851, #27635, .T. ) ;
#9004=AXIS2_PLACEMENT_3D ( 'NONE', #2330, #17589, #6863 ) ;
#9011=B_SPLINE_CURVE_WITH_KNOTS ( 'NONE', 3,
 ( #3282, #16303, #7253, #24905, #14192, #13751, #2858, #22794, #11496, #3418 ),
 .UNSPECIFIED., .F., .F.,
 ( 4, 2, 2, 2, 4 ),
 ( 0.000000000000000000, 0.2500000000000000000, 0.5000000000000000000, 0.7500000000000000000, 1.000000000000000000 ),
 .UNSPECIFIED. ) ;
#9019=ORIENTED_EDGE ( 'NONE', *, *, #26613, .T. ) ;
#9035=CARTESIAN_POINT ( 'NONE',  ( 0.000000000000000000, 0.000000000000000000, 0.09685039370078740717 ) ) ;
#9050=ORIENTED_EDGE ( 'NONE', *, *, #5186, .F. ) ;
#9062=CARTESIAN_POINT ( 'NONE',  ( -0.5383572925356228112, -0.3100567972183445042, 0.2574803149606298969 ) ) ;
#9069=DIRECTION ( 'NONE',  ( 0.000000000000000000, 0.000000000000000000, 1.000000000000000000 ) ) ;
#9085=LINE ( 'NONE', #761, #4626 ) ;
#9091=DIRECTION ( 'NONE',  ( 0.000000000000000000, 0.000000000000000000, 1.000000000000000000 ) ) ;
#9099=EDGE_CURVE ( 'NONE', #25691, #18857, #13634, .T. ) ;
#9112=VECTOR ( 'NONE', #6719, 39.37007874015748143 ) ;
#9143=CARTESIAN_POINT ( 'NONE',  ( -0.4009292313423786780, -0.2321359940675791766, 0.2048502514806590791 ) ) ;
#9180=ADVANCED_FACE ( 'NONE', ( #16661 ), #16805, .F. ) ;
#9201=DIRECTION ( 'NONE',  ( 0.000000000000000000, 0.000000000000000000, 1.000000000000000000 ) ) ;
#9204=CIRCLE ( 'NONE', #2890, 0.5007874015748031704 ) ;
#9205=FACE_BOUND ( 'NONE', #20169, .T. ) ;
#9215=FACE_OUTER_BOUND ( 'NONE', #14839, .T. ) ;
#9216=VERTEX_POINT ( 'NONE', #8052 ) ;
#9227=FACE_OUTER_BOUND ( 'NONE', #8847, .T. ) ;
#9230=DIRECTION ( 'NONE',  ( 0.000000000000000000, 0.000000000000000000, -1.000000000000000000 ) ) ;
#9231=EDGE_CURVE ( 'NONE', #1804, #8934, #11449, .T. ) ;
#9234=CARTESIAN_POINT ( 'NONE',  ( -0.0002199787722624904878, 0.6212598425196850238, 0.2574827755769819038 ) ) ;
#9254=VERTEX_POINT ( 'NONE', #20895 ) ;
#9277=CARTESIAN_POINT ( 'NONE',  ( -0.3214446924536846772, 0.3840069416942866742, 0.2574803149606298969 ) ) ;
#9285=EDGE_LOOP ( 'NONE', ( #23979, #22439, #19635, #1175 ) ) ;
#9294=DIRECTION ( 'NONE',  ( 0.000000000000000000, 0.000000000000000000, -1.000000000000000000 ) ) ;
#9297=DIRECTION ( 'NONE',  ( 0.000000000000000000, 0.000000000000000000, 1.000000000000000000 ) ) ;
#9322=ORIENTED_EDGE ( 'NONE', *, *, #5056, .T. ) ;
#9324=CARTESIAN_POINT ( 'NONE',  ( 0.4334967711386992772, -0.2507361369899905879, 0.2574819596263889787 ) ) ;
#9328=AXIS2_PLACEMENT_3D ( 'NONE', #23556, #13207, #19716 ) ;
#9330=CARTESIAN_POINT ( 'NONE',  ( -0.4931105264837953306, 0.08735026989778622852, 0.2574819596263889787 ) ) ;
#9336=CARTESIAN_POINT ( 'NONE',  ( 0.6118597084614586512, 0.1076640027107649555, 0.2574827755769819038 ) ) ;
#9343=CARTESIAN_POINT ( 'NONE',  ( -0.5579526598170320151, -0.3213561723284472094, 0.2359405056215991836 ) ) ;
#9348=CARTESIAN_POINT ( 'NONE',  ( 0.000000000000000000, 0.000000000000000000, 0.1771653543307086520 ) ) ;
#9355=EDGE_LOOP ( 'NONE', ( #22610, #9386 ) ) ;
#9358=CARTESIAN_POINT ( 'NONE',  ( -0.4930758245789425009, 0.08754571829529331217, 0.09685039370078740717 ) ) ;
#9386=ORIENTED_EDGE ( 'NONE', *, *, #7701, .T. ) ;
#9393=VERTEX_POINT ( 'NONE', #20400 ) ;
#9396=FACE_OUTER_BOUND ( 'NONE', #22391, .T. ) ;
#9398=DIRECTION ( 'NONE',  ( 1.000000000000000000, 0.000000000000000000, 0.000000000000000000 ) ) ;
#9414=B_SPLINE_CURVE_WITH_KNOTS ( 'NONE', 3,
 ( #6550, #19258, #15326, #17413, #8793, #13166 ),
 .UNSPECIFIED., .F., .F.,
 ( 4, 2, 4 ),
 ( 0.9031406754215579591, 0.9046454396443720514, 0.9061502038671850334 ),
 .UNSPECIFIED. ) ;
#9436=CARTESIAN_POINT ( 'NONE',  ( -0.0006615832606325197825, 0.6212594902576319411, 0.09685039370078740717 ) ) ;
#9437=CARTESIAN_POINT ( 'NONE',  ( -0.4216473064060453635, -0.2427620699883266953, 0.2467937633103768902 ) ) ;
#9457=EDGE_CURVE ( 'NONE', #16353, #11971, #15481, .T. ) ;
#9461=CARTESIAN_POINT ( 'NONE',  ( -0.4858607088160732390, -0.2805118110236220486, 0.07676968503937006694 ) ) ;
#9465=DIRECTION ( 'NONE',  ( 0.000000000000000000, 0.000000000000000000, 1.000000000000000000 ) ) ;
#9472=VERTEX_POINT ( 'NONE', #9803 ) ;
#9487=FACE_BOUND ( 'NONE', #27478, .T. ) ;
#9488=CARTESIAN_POINT ( 'NONE',  ( -0.5491102354219716819, -0.3162573801175062038, 0.1061598535667389875 ) ) ;
#9497=AXIS2_PLACEMENT_3D ( 'NONE', #27644, #8288, #10530 ) ;
#9515=CIRCLE ( 'NONE', #22156, 0.6212598425196850238 ) ;
#9545=DIRECTION ( 'NONE',  ( 0.000000000000000000, 0.000000000000000000, -1.000000000000000000 ) ) ;
#9561=CARTESIAN_POINT ( 'NONE',  ( 0.2195865873864355222, -0.6052790189103738339, 0.2359405056189624594 ) ) ;
#9586=EDGE_LOOP ( 'NONE', ( #22344, #9756, #14033, #23346 ) ) ;
#9587=DIRECTION ( 'NONE',  ( 0.000000000000000000, 1.000000000000000000, 0.000000000000000000 ) ) ;
#9594=CIRCLE ( 'NONE', #20437, 0.7283464566929134243 ) ;
#9599=ORIENTED_EDGE ( 'NONE', *, *, #17818, .F. ) ;
#9631=CARTESIAN_POINT ( 'NONE',  ( 0.1710938124795997883, -0.4706537664821763833, 0.2574827755769819038 ) ) ;
#9632=DIRECTION ( 'NONE',  ( 0.8660254037844385966, -0.5000000000000003331, 0.000000000000000000 ) ) ;
#9654=DIRECTION ( 'NONE',  ( 0.000000000000000000, 0.000000000000000000, 1.000000000000000000 ) ) ;
#9662=B_SPLINE_CURVE_WITH_KNOTS ( 'NONE', 3,
 ( #7490, #25250, #16117, #12396, #23144, #10410, #14687, #21155, #16636, #27524 ),
 .UNSPECIFIED., .F., .F.,
 ( 4, 2, 2, 2, 4 ),
 ( 0.000000000000000000, 0.2500000000000001110, 0.5000000000000002220, 0.7500000000000003331, 1.000000000000000000 ),
 .UNSPECIFIED. ) ;
#9717=CIRCLE ( 'NONE', #25499, 0.1003956692913385712 ) ;
#9726=ORIENTED_EDGE ( 'NONE', *, *, #19797, .T. ) ;
#9752=DIRECTION ( 'NONE',  ( 0.000000000000000000, 0.000000000000000000, 1.000000000000000000 ) ) ;
#9756=ORIENTED_EDGE ( 'NONE', *, *, #27758, .F. ) ;
#9757=EDGE_CURVE ( 'NONE', #11845, #21446, #204, .T. ) ;
#9764=CARTESIAN_POINT ( 'NONE',  ( -0.1570092758121678089, -0.4330450457732858416, 0.1771653543307084855 ) ) ;
#9773=AXIS2_PLACEMENT_3D ( 'NONE', #17443, #9091, #25926 ) ;
#9775=EDGE_LOOP ( 'NONE', ( #24301, #6819, #12896, #2814, #4943, #11835, #5030, #17505, #18697, #22390, #14010, #23296, #25147 ) ) ;
#9776=CARTESIAN_POINT ( 'NONE',  ( -4.821444091131312140E-17, -0.3937007874015748254, 0.1771653543307086520 ) ) ;
#9787=ORIENTED_EDGE ( 'NONE', *, *, #23893, .T. ) ;
#9803=CARTESIAN_POINT ( 'NONE',  ( 0.2118615749922464486, -0.5840192333899535404, 0.2574803149606298969 ) ) ;
#9808=AXIS2_PLACEMENT_3D ( 'NONE', #25301, #3829, #5963 ) ;
#9844=CARTESIAN_POINT ( 'NONE',  ( 0.0006615832605804723319, 0.6212594902576319411, 0.2574803149606298969 ) ) ;
#9848=CARTESIAN_POINT ( 'NONE',  ( 0.3131893444329049703, 0.3723335979450146382, 0.2467937633107637474 ) ) ;
#9885=CARTESIAN_POINT ( 'NONE',  ( 0.2122766679520079192, -0.5838685267775929333, 0.2574827755769819038 ) ) ;
#9890=EDGE_LOOP ( 'NONE', ( #4341, #4015 ) ) ;
#9894=DIRECTION ( 'NONE',  ( 0.000000000000000000, 0.000000000000000000, 1.000000000000000000 ) ) ;
#9906=CARTESIAN_POINT ( 'NONE',  ( -0.6514872030428984218, 0.1141809932450963266, 0.1926811207670676152 ) ) ;
#9908=DIRECTION ( 'NONE',  ( 1.000000000000000000, 0.000000000000000000, 0.000000000000000000 ) ) ;
#9932=FACE_OUTER_BOUND ( 'NONE', #24940, .T. ) ;
#9935=DIRECTION ( 'NONE',  ( 0.000000000000000000, 0.000000000000000000, 1.000000000000000000 ) ) ;
#9942=B_SPLINE_CURVE_WITH_KNOTS ( 'NONE', 3,
 ( #11618, #3131, #20241, #22643, #26448, #13884 ),
 .UNSPECIFIED., .F., .F.,
 ( 4, 2, 4 ),
 ( 0.9031406754215579591, 0.9046454396443720514, 0.9061502038671860326 ),
 .UNSPECIFIED. ) ;
#9949=TOROIDAL_SURFACE ( 'NONE', #2273, 0.5610236220472440971, 0.1003937007874015908 ) ;
#9955=DIRECTION ( 'NONE',  ( 0.000000000000000000, 0.000000000000000000, 1.000000000000000000 ) ) ;
#9961=ORIENTED_EDGE ( 'NONE', *, *, #13512, .T. ) ;
#9971=FACE_BOUND ( 'NONE', #9285, .T. ) ;
#9989=ORIENTED_EDGE ( 'NONE', *, *, #27181, .F. ) ;
#10019=ORIENTED_EDGE ( 'NONE', *, *, #22804, .T. ) ;
#10025=CARTESIAN_POINT ( 'NONE',  ( 0.2118615749922464486, -0.5840192333899535404, 0.2574803149606298969 ) ) ;
#10037=ADVANCED_FACE ( 'NONE', ( #17814 ), #1958, .F. ) ;
#10043=CARTESIAN_POINT ( 'NONE',  ( 3.644242538420618632E-18, 0.5007874015748032814, 0.09684793308443545579 ) ) ;
#10058=VERTEX_POINT ( 'NONE', #15715 ) ;
#10061=DIRECTION ( 'NONE',  ( 0.000000000000000000, 0.000000000000000000, 1.000000000000000000 ) ) ;
#10070=FACE_OUTER_BOUND ( 'NONE', #2427, .T. ) ;
#10077=CARTESIAN_POINT ( 'NONE',  ( -0.2126900928101220500, -0.5837180524351338606, 0.2574827755769819038 ) ) ;
#10087=EDGE_CURVE ( 'NONE', #27463, #6066, #26908, .T. ) ;
#10095=DIRECTION ( 'NONE',  ( 0.000000000000000000, 0.000000000000000000, 1.000000000000000000 ) ) ;
#10109=ORIENTED_EDGE ( 'NONE', *, *, #23236, .T. ) ;
#10123=DIRECTION ( 'NONE',  ( 0.000000000000000000, 1.000000000000000000, 0.000000000000000000 ) ) ;
#10129=CARTESIAN_POINT ( 'NONE',  ( 0.3988311005572732215, 0.4763376377695315300, 0.2574803149606298969 ) ) ;
#10150=CARTESIAN_POINT ( 'NONE',  ( -0.3217486617182078734, 0.3837523410419874659, 0.2574827755769819038 ) ) ;
#10165=CARTESIAN_POINT ( 'NONE',  ( 6.147461752294700483E-18, 0.5610236220472440971, 0.2775610236220472093 ) ) ;
#10166=DIRECTION ( 'NONE',  ( 0.000000000000000000, 0.000000000000000000, 1.000000000000000000 ) ) ;
#10168=ORIENTED_EDGE ( 'NONE', *, *, #19797, .F. ) ;
#10171=FACE_OUTER_BOUND ( 'NONE', #10325, .T. ) ;
#10174=ORIENTED_EDGE ( 'NONE', *, *, #18912, .T. ) ;
#10184=FACE_BOUND ( 'NONE', #16326, .T. ) ;
#10186=CARTESIAN_POINT ( 'NONE',  ( 0.4930758245789425009, 0.08754571829529310401, 0.09685039370078740717 ) ) ;
#10194=EDGE_CURVE ( 'NONE', #6124, #5913, #14842, .T. ) ;
#10201=VERTEX_POINT ( 'NONE', #14597 ) ;
#10219=B_SPLINE_CURVE_WITH_KNOTS ( 'NONE', 3,
 ( #12277, #21184, #10150, #18765, #23171, #3805 ),
 .UNSPECIFIED., .F., .F.,
 ( 4, 2, 4 ),
 ( 0.9031406754215579591, 0.9046454396443720514, 0.9061502038671860326 ),
 .UNSPECIFIED. ) ;
#10226=( NAMED_UNIT ( * ) SI_UNIT ( $, .STERADIAN. ) SOLID_ANGLE_UNIT ( ) ) ;
#10232=CARTESIAN_POINT ( 'NONE',  ( 0.2268599607420258568, -0.6212949646986238861, 0.1926811207639263224 ) ) ;
#10238=CARTESIAN_POINT ( 'NONE',  ( -0.3606190329934327310, 0.4297690281277732338, 0.2775610236220472093 ) ) ;
#10240=ORIENTED_EDGE ( 'NONE', *, *, #15648, .F. ) ;
#10241=ORIENTED_EDGE ( 'NONE', *, *, #8485, .F. ) ;
#10254=DIRECTION ( 'NONE',  ( 1.000000000000000000, 0.000000000000000000, 0.000000000000000000 ) ) ;
#10267=EDGE_CURVE ( 'NONE', #20711, #15905, #5523, .T. ) ;
#10272=CARTESIAN_POINT ( 'NONE',  ( -0.4233199042382427835, 0.5034331896112764770, 0.2081850588231654031 ) ) ;
#10284=DIRECTION ( 'NONE',  ( 0.7660444431189780135, 0.6427876096865392519, 0.000000000000000000 ) ) ;
#10286=CARTESIAN_POINT ( 'NONE',  ( 0.1658556822987644341, -0.4573967274800467275, 0.2467937633379344575 ) ) ;
#10290=DIRECTION ( 'NONE',  ( 0.000000000000000000, 1.000000000000000000, 0.000000000000000000 ) ) ;
#10300=EDGE_CURVE ( 'NONE', #6477, #17148, #19514, .T. ) ;
#10301=CARTESIAN_POINT ( 'NONE',  ( 0.5383572925355708527, -0.3100567972184350429, 0.2574803149606298969 ) ) ;
#10304=CARTESIAN_POINT ( 'NONE',  ( 0.1589886963210821458, -0.4351482077929094694, 0.2048502515443846317 ) ) ;
#10305=ORIENTED_EDGE ( 'NONE', *, *, #3152, .T. ) ;
#10308=CARTESIAN_POINT ( 'NONE',  ( 0.000000000000000000, 0.000000000000000000, 0.1771653543307086520 ) ) ;
#10316=AXIS2_PLACEMENT_3D ( 'NONE', #24959, #22999, #5618 ) ;
#10320=EDGE_CURVE ( 'NONE', #24998, #13907, #377, .T. ) ;
#10321=CARTESIAN_POINT ( 'NONE',  ( -0.1714649452450071054, -0.4705186852026070898, 0.2574827755769819038 ) ) ;
#10324=PRODUCT_DEFINITION ( 'UNKNOWN', '', #13832, #8531 ) ;
#10325=EDGE_LOOP ( 'NONE', ( #17826, #11809, #8130, #21397, #27271 ) ) ;
#10334=SPHERICAL_SURFACE ( 'NONE', #24090, 0.1003956692913385851 ) ;
#10338=AXIS2_PLACEMENT_3D ( 'NONE', #19787, #11303, #21638 ) ;
#10359=AXIS2_PLACEMENT_3D ( 'NONE', #6590, #6445, #12931 ) ;
#10362=ORIENTED_EDGE ( 'NONE', *, *, #19686, .F. ) ;
#10363=ADVANCED_FACE ( 'NONE', ( #12121, #16229 ), #5919, .T. ) ;
#10369=CARTESIAN_POINT ( 'NONE',  ( 0.1918813796216842782, -0.5271897577243779276, 0.1771653543307086520 ) ) ;
#10374=AXIS2_PLACEMENT_3D ( 'NONE', #27120, #24982, #25270 ) ;
#10410=CARTESIAN_POINT ( 'NONE',  ( -0.2268599607415389408, -0.6212949646972618645, 0.1616495878881323567 ) ) ;
#10424=ORIENTED_EDGE ( 'NONE', *, *, #22013, .T. ) ;
#10451=CARTESIAN_POINT ( 'NONE',  ( 0.4932136069632150344, 0.08676634416061969335, 0.09684793308443523374 ) ) ;
#10452=DIRECTION ( 'NONE',  ( 1.000000000000000000, 0.000000000000000000, 0.000000000000000000 ) ) ;
#10461=EDGE_CURVE ( 'NONE', #16455, #3818, #22200, .T. ) ;
#10466=EDGE_LOOP ( 'NONE', ( #982, #3793, #3347, #14268, #3214, #4617, #22933, #25259, #23868, #23974, #13954, #20270, #6173 ) ) ;
#10468=CARTESIAN_POINT ( 'NONE',  ( 0.000000000000000000, 0.000000000000000000, 0.1771653543307086520 ) ) ;
#10469=CARTESIAN_POINT ( 'NONE',  ( 0.0005789383928842625369, 0.4762008496972124916, 0.2330651857772763624 ) ) ;
#10488=ADVANCED_FACE ( 'NONE', ( #23579, #8721 ), #17342, .T. ) ;
#10489=CARTESIAN_POINT ( 'NONE',  ( 0.000000000000000000, 0.000000000000000000, 0.04842519685039370358 ) ) ;
#10513=B_SPLINE_CURVE_WITH_KNOTS ( 'NONE', 3,
 ( #1987, #16973, #12721, #14880, #19079, #25588 ),
 .UNSPECIFIED., .F., .F.,
 ( 4, 2, 4 ),
 ( 0.000000000000000000, 0.2500000000000000000, 0.5000000000000000000 ),
 .UNSPECIFIED. ) ;
#10519=ORIENTED_EDGE ( 'NONE', *, *, #23397, .F. ) ;
#10524=CARTESIAN_POINT ( 'NONE',  ( -0.2118615749922468650, -0.5840192333899535404, 0.2574803149606298969 ) ) ;
#10530=DIRECTION ( 'NONE',  ( -1.000000000000000000, 1.224646799147346305E-16, 0.000000000000000000 ) ) ;
#10551=CARTESIAN_POINT ( 'NONE',  ( 0.4930758245789425009, 0.08754571829529310401, 0.2574803149606298969 ) ) ;
#10554=EDGE_CURVE ( 'NONE', #22901, #15797, #26259, .T. ) ;
#10569=CARTESIAN_POINT ( 'NONE',  ( 0.1570092758121686138, -0.4330450457732857861, 0.1903859678454303539 ) ) ;
#10608=ORIENTED_EDGE ( 'NONE', *, *, #21762, .F. ) ;
#10618=CIRCLE ( 'NONE', #19198, 0.3937007874015748254 ) ;
#10631=CARTESIAN_POINT ( 'NONE',  ( 0.4222761783103636257, 0.5043089796496124100, 0.1461456498321524189 ) ) ;
#10639=DIRECTION ( 'NONE',  ( 1.000000000000000000, 0.000000000000000000, 0.000000000000000000 ) ) ;
#10643=DIRECTION ( 'NONE',  ( -1.000000000000000000, 1.224646799147353454E-16, 0.000000000000000000 ) ) ;
#10671=CIRCLE ( 'NONE', #18333, 0.01181102362204724046 ) ;
#10680=CARTESIAN_POINT ( 'NONE',  ( -0.6118978891064095205, 0.1074467966294590654, 0.2574819594177531479 ) ) ;
#10694=COLOUR_RGB ( '', 0.08235294, 0.09019608, 0.10196078) ;
#10748=CARTESIAN_POINT ( 'NONE',  ( 0.5383572925355968319, -0.3100567972183901899, 0.09685039370078740717 ) ) ;
#10760=CARTESIAN_POINT ( 'NONE',  ( 0.000000000000000000, 0.000000000000000000, 0.3543307086614173040 ) ) ;
#10769=CARTESIAN_POINT ( 'NONE',  ( -0.4210617728879400001, -0.2437762437905965363, 0.1075369453512742129 ) ) ;
#10783=ORIENTED_EDGE ( 'NONE', *, *, #14264, .T. ) ;
#10791=AXIS2_PLACEMENT_3D ( 'NONE', #27519, #27231, #8165 ) ;
#10844=ORIENTED_EDGE ( 'NONE', *, *, #6615, .F. ) ;
#10854=CARTESIAN_POINT ( 'NONE',  ( 0.000000000000000000, 0.000000000000000000, 0.09685039370078740717 ) ) ;
#10855=CARTESIAN_POINT ( 'NONE',  ( 0.1579154690117922366, -0.4355388305902855306, 0.2048502515516587574 ) ) ;
#10867=CARTESIAN_POINT ( 'NONE',  ( -0.3056525133678795747, 0.3651631491437063448, 0.2330651857751106226 ) ) ;
#10869=VERTEX_POINT ( 'NONE', #6019 ) ;
#10870=EDGE_CURVE ( 'NONE', #25476, #13715, #11056, .T. ) ;
#10880=FACE_OUTER_BOUND ( 'NONE', #12086, .T. ) ;
#10890=AXIS2_PLACEMENT_3D ( 'NONE', #22947, #16722, #13902 ) ;
#10903=DIRECTION ( 'NONE',  ( 0.000000000000000000, 0.000000000000000000, 1.000000000000000000 ) ) ;
#10905=CARTESIAN_POINT ( 'NONE',  ( 0.000000000000000000, 0.000000000000000000, 0.2574803149606298969 ) ) ;
#10907=EDGE_CURVE ( 'NONE', #15613, #4851, #2288, .T. ) ;
#10914=EDGE_CURVE ( 'NONE', #21446, #4739, #9085, .T. ) ;
#10922=ORIENTED_EDGE ( 'NONE', *, *, #18912, .F. ) ;
#10926=ADVANCED_FACE ( 'NONE', ( #26055 ), #19834, .F. ) ;
#10939=ADVANCED_FACE ( 'NONE', ( #9215 ), #13462, .T. ) ;
#10948=CARTESIAN_POINT ( 'NONE',  ( -0.6117062799105531523, 0.1085321106658068829, 0.2574803149606298969 ) ) ;
#10958=CARTESIAN_POINT ( 'NONE',  ( 0.2982299571069384481, 0.3545282230944422630, 0.1494804571808522331 ) ) ;
#10980=CARTESIAN_POINT ( 'NONE',  ( 0.000000000000000000, 0.5610236220472440971, 0.1771653543307086520 ) ) ;
#10987=CARTESIAN_POINT ( 'NONE',  ( 0.6118597084614606496, 0.1076640027107480246, 0.09684793308443542803 ) ) ;
#11007=VERTEX_POINT ( 'NONE', #27036 ) ;
#11028=B_SPLINE_CURVE_WITH_KNOTS ( 'NONE', 3,
 ( #4253, #4389, #60, #12858, #8625, #17244 ),
 .UNSPECIFIED., .F., .F.,
 ( 4, 2, 4 ),
 ( 0.3000437156586439613, 0.3015484798814569989, 0.3030532441042709801 ),
 .UNSPECIFIED. ) ;
#11030=CARTESIAN_POINT ( 'NONE',  ( -0.1714649452450071054, -0.4705186852026070898, 0.09684793308443542803 ) ) ;
#11052=VERTEX_POINT ( 'NONE', #22648 ) ;
#11055=AXIS2_PLACEMENT_3D ( 'NONE', #15407, #21882, #1412 ) ;
#11056=B_SPLINE_CURVE_WITH_KNOTS ( 'NONE', 3,
 ( #6571, #19421, #23403, #27629, #15196, #10232, #23677, #18846, #27488, #12509 ),
 .UNSPECIFIED., .F., .F.,
 ( 4, 2, 2, 2, 4 ),
 ( 0.000000000000000000, 0.2500000000000002776, 0.5000000000000005551, 0.7500000000000002220, 1.000000000000000000 ),
 .UNSPECIFIED. ) ;
#11059=CARTESIAN_POINT ( 'NONE',  ( -0.6118978891064172920, 0.1074467966294249954, 0.09684874924366436433 ) ) ;
#11088=ORIENTED_EDGE ( 'NONE', *, *, #6634, .T. ) ;
#11112=AXIS2_PLACEMENT_3D ( 'NONE', #10308, #6366, #6102 ) ;
#11119=CARTESIAN_POINT ( 'NONE',  ( -0.0006615832605804723319, 0.6212594902576319411, 0.2574803149606298969 ) ) ;
#11123=ORIENTED_EDGE ( 'NONE', *, *, #746, .F. ) ;
#11129=B_SPLINE_CURVE_WITH_KNOTS ( 'NONE', 3,
 ( #13477, #22107, #13077, #10958, #19582, #261 ),
 .UNSPECIFIED., .F., .F.,
 ( 4, 2, 4 ),
 ( 0.000000000000000000, 0.2500000000000000000, 0.5000000000000000000 ),
 .UNSPECIFIED. ) ;
#11144=( LENGTH_UNIT ( ) NAMED_UNIT ( * ) SI_UNIT ( $, .METRE. ) ) ;
#11159=CARTESIAN_POINT ( 'NONE',  ( 0.2956505864974370845, 0.3532288989643546095, 0.1903859677965938912 ) ) ;
#11177=ORIENTED_EDGE ( 'NONE', *, *, #23690, .F. ) ;
#11191=CARTESIAN_POINT ( 'NONE',  ( 0.000000000000000000, 0.000000000000000000, 0.2574803149606298969 ) ) ;
#11194=ORIENTED_EDGE ( 'NONE', *, *, #129, .T. ) ;
#11195=AXIS2_PLACEMENT_3D ( 'NONE', #21204, #23047, #10452 ) ;
#11198=CARTESIAN_POINT ( 'NONE',  ( -0.3937007874015748254, 4.893765752498281459E-17, 0.3425196850393700809 ) ) ;
#11211=CARTESIAN_POINT ( 'NONE',  ( 0.000000000000000000, 0.000000000000000000, 0.3059055118110236560 ) ) ;
#11221=CIRCLE ( 'NONE', #6260, 0.6212598425196850238 ) ;
#11228=CARTESIAN_POINT ( 'NONE',  ( 0.6476458834277908361, 0.1148891961917465482, 0.2081850588316230821 ) ) ;
#11239=ORIENTED_EDGE ( 'NONE', *, *, #15878, .T. ) ;
#11242=CARTESIAN_POINT ( 'NONE',  ( -0.6476458834271923148, 0.1148891961916498478, 0.1461456498280682970 ) ) ;
#11247=EDGE_LOOP ( 'NONE', ( #21822, #17189, #9787, #12456 ) ) ;
#11278=DIRECTION ( 'NONE',  ( 0.000000000000000000, 1.000000000000000000, 0.000000000000000000 ) ) ;
#11281=ORIENTED_EDGE ( 'NONE', *, *, #19826, .T. ) ;
#11297=DIRECTION ( 'NONE',  ( 0.000000000000000000, 1.000000000000000000, 0.000000000000000000 ) ) ;
#11303=DIRECTION ( 'NONE',  ( -0.8660254037844388186, -0.4999999999999997780, 0.000000000000000000 ) ) ;
#11319=EDGE_CURVE ( 'NONE', #17345, #22917, #9594, .T. ) ;
#11322=EDGE_CURVE ( 'NONE', #11971, #25691, #3277, .T. ) ;
#11350=CARTESIAN_POINT ( 'NONE',  ( -0.0006737210091418004447, 0.6438792636756986987, 0.1183902030408860162 ) ) ;
#11359=VERTEX_POINT ( 'NONE', #3965 ) ;
#11361=DIRECTION ( 'NONE',  ( -0.8660254037844385966, -0.5000000000000002220, 0.000000000000000000 ) ) ;
#11418=EDGE_LOOP ( 'NONE', ( #11948, #27000, #19212, #20771 ) ) ;
#11429=CARTESIAN_POINT ( 'NONE',  ( 0.4932478747986535628, 0.08657132889677619791, 0.2574819596263889787 ) ) ;
#11449=B_SPLINE_CURVE_WITH_KNOTS ( 'NONE', 3,
 ( #3503, #5359, #23166, #22592, #18762, #27122 ),
 .UNSPECIFIED., .F., .F.,
 ( 4, 2, 4 ),
 ( 0.3108507187342950395, 0.3125269569790680158, 0.3142031952238389936 ),
 .UNSPECIFIED. ) ;
#11455=VERTEX_POINT ( 'NONE', #16793 ) ;
#11459=CARTESIAN_POINT ( 'NONE',  ( 0.000000000000000000, 0.000000000000000000, 0.04842519685039370358 ) ) ;
#11464=DIRECTION ( 'NONE',  ( 1.000000000000000000, 0.000000000000000000, 0.000000000000000000 ) ) ;
#11485=CARTESIAN_POINT ( 'NONE',  ( -0.5731455175601024576, -0.3301167833454110578, 0.1926811207745849075 ) ) ;
#11496=CARTESIAN_POINT ( 'NONE',  ( 0.5491102354215032788, -0.3162573801172474663, 0.2481708550950798842 ) ) ;
#11502=CARTESIAN_POINT ( 'NONE',  ( 0.3998447049182496382, 0.4754871227240771714, 0.09685039370078740717 ) ) ;
#11514=CARTESIAN_POINT ( 'NONE',  ( 0.3606190329934327310, 0.4297690281277732338, 0.1771653543307086520 ) ) ;
#11522=ORIENTED_EDGE ( 'NONE', *, *, #3428, .F. ) ;
#11530=CYLINDRICAL_SURFACE ( 'NONE', #26314, 0.5007874015748031704 ) ;
#11588=AXIS2_PLACEMENT_3D ( 'NONE', #5229, #3665, #7923 ) ;
#11597=CARTESIAN_POINT ( 'NONE',  ( -0.2243259791918627288, -0.6183223858019056829, 0.1461456498332554532 ) ) ;
#11611=DIRECTION ( 'NONE',  ( 0.000000000000000000, 0.000000000000000000, 1.000000000000000000 ) ) ;
#11618=CARTESIAN_POINT ( 'NONE',  ( 0.3223547283257516272, 0.3832433309296771617, 0.2574803149606298969 ) ) ;
#11634=EDGE_LOOP ( 'NONE', ( #7052, #8787, #14488, #27392 ) ) ;
#11636=EDGE_CURVE ( 'NONE', #27798, #478, #16796, .T. ) ;
#11649=EDGE_LOOP ( 'NONE', ( #1319, #15798 ) ) ;
#11680=CARTESIAN_POINT ( 'NONE',  ( 0.6478824768887737617, 0.1135474080050588724, 0.1461456498333656429 ) ) ;
#11687=DIRECTION ( 'NONE',  ( -0.9848077530122077983, 0.1736481776669313304, 0.000000000000000000 ) ) ;
#11709=CARTESIAN_POINT ( 'NONE',  ( 0.4932821129636645874, 0.08637579872942321990, 0.2574803149606298969 ) ) ;
#11712=CARTESIAN_POINT ( 'NONE',  ( 0.000000000000000000, 0.000000000000000000, 0.1771653543307086520 ) ) ;
#11715=CARTESIAN_POINT ( 'NONE',  ( -0.4246272423000664875, 0.5071139714518992925, 0.1616495878844767808 ) ) ;
#11717=B_SPLINE_CURVE_WITH_KNOTS ( 'NONE', 3,
 ( #12921, #17174, #2052, #8415, #27352, #4181, #12789, #25788, #8555, #8282 ),
 .UNSPECIFIED., .F., .F.,
 ( 4, 2, 2, 2, 4 ),
 ( 0.000000000000000000, 0.2500000000000000000, 0.5000000000000000000, 0.7500000000000000000, 1.000000000000000000 ),
 .UNSPECIFIED. ) ;
#11724=DIRECTION ( 'NONE',  ( -0.9848077530122082424, -0.1736481776669300259, 0.000000000000000000 ) ) ;
#11735=VERTEX_POINT ( 'NONE', #26635 ) ;
#11746=ORIENTED_EDGE ( 'NONE', *, *, #21955, .F. ) ;
#11765=CARTESIAN_POINT ( 'NONE',  ( -7.608238775805210269E-17, -0.6212598425196850238, 0.04842519685039370358 ) ) ;
#11771=AXIS2_PLACEMENT_3D ( 'NONE', #23551, #20991, #3753 ) ;
#11775=CARTESIAN_POINT ( 'NONE',  ( -0.1718374205099799101, -0.4703827404237102550, 0.09685039370078740717 ) ) ;
#11779=VERTEX_POINT ( 'NONE', #7291 ) ;
#11809=ORIENTED_EDGE ( 'NONE', *, *, #6996, .T. ) ;
#11820=DIRECTION ( 'NONE',  ( 0.000000000000000000, -1.000000000000000000, 0.000000000000000000 ) ) ;
#11826=CARTESIAN_POINT ( 'NONE',  ( 0.3214446924536846772, 0.3840069416942866742, 0.09685039370078740717 ) ) ;
#11835=ORIENTED_EDGE ( 'NONE', *, *, #5501, .T. ) ;
#11844=CARTESIAN_POINT ( 'NONE',  ( 0.4338922498494567348, -0.2500511477696476526, 0.09684874903502814492 ) ) ;
#11845=VERTEX_POINT ( 'NONE', #10524 ) ;
#11870=ORIENTED_EDGE ( 'NONE', *, *, #14644, .T. ) ;
#11872=ORIENTED_EDGE ( 'NONE', *, *, #10320, .T. ) ;
#11875=DIRECTION ( 'NONE',  ( 0.000000000000000000, 1.000000000000000000, 0.000000000000000000 ) ) ;
#11876=AXIS2_PLACEMENT_3D ( 'NONE', #13113, #19626, #2235 ) ;
#11878=VERTEX_POINT ( 'NONE', #16751 ) ;
#11879=DIRECTION ( 'NONE',  ( 0.000000000000000000, 1.000000000000000000, 0.000000000000000000 ) ) ;
#11900=VERTEX_POINT ( 'NONE', #10238 ) ;
#11904=VERTEX_POINT ( 'NONE', #18853 ) ;
#11909=ORIENTED_EDGE ( 'NONE', *, *, #2419, .T. ) ;
#11933=ORIENTED_EDGE ( 'NONE', *, *, #18967, .T. ) ;
#11943=ORIENTED_EDGE ( 'NONE', *, *, #4096, .T. ) ;
#11948=ORIENTED_EDGE ( 'NONE', *, *, #9231, .F. ) ;
#11969=CARTESIAN_POINT ( 'NONE',  ( 0.5382469622846756119, -0.3102483656526354716, 0.2574819594177531479 ) ) ;
#11971=VERTEX_POINT ( 'NONE', #20660 ) ;
#11974=ADVANCED_FACE ( 'NONE', ( #897 ), #18976, .F. ) ;
#11976=FACE_BOUND ( 'NONE', #25512, .T. ) ;
#11981=CARTESIAN_POINT ( 'NONE',  ( 0.1718374205099799101, -0.4703827404237102550, 0.09685039370078740717 ) ) ;
#11984=CARTESIAN_POINT ( 'NONE',  ( 0.000000000000000000, 0.3937007874015748254, 0.01181102362204724393 ) ) ;
#12000=ADVANCED_FACE ( 'NONE', ( #22638, #16151 ), #26583, .T. ) ;
#12014=EDGE_CURVE ( 'NONE', #13235, #8311, #1822, .T. ) ;
#12019=CARTESIAN_POINT ( 'NONE',  ( 0.000000000000000000, 0.000000000000000000, 0.09685039370078740717 ) ) ;
#12023=ORIENTED_EDGE ( 'NONE', *, *, #23619, .F. ) ;
#12032=CARTESIAN_POINT ( 'NONE',  ( 0.2131049448083992270, -0.5835666837866889667, 0.09685039370078740717 ) ) ;
#12041=DIRECTION ( 'NONE',  ( -1.000000000000000000, 1.224646799147353454E-16, 0.000000000000000000 ) ) ;
#12049=DIRECTION ( 'NONE',  ( 0.000000000000000000, -1.000000000000000000, 0.000000000000000000 ) ) ;
#12056=CARTESIAN_POINT ( 'NONE',  ( -0.4932136069632142017, 0.08676634416062008193, 0.09684793308443542803 ) ) ;
#12060=AXIS2_PLACEMENT_3D ( 'NONE', #15085, #25530, #6320 ) ;
#12062=DIRECTION ( 'NONE',  ( 0.000000000000000000, 0.000000000000000000, 1.000000000000000000 ) ) ;
#12076=DIRECTION ( 'NONE',  ( 0.000000000000000000, 1.000000000000000000, 0.000000000000000000 ) ) ;
#12079=CARTESIAN_POINT ( 'NONE',  ( 0.3996755081322992398, 0.4756294029998582307, 0.09684874924366436433 ) ) ;
#12086=EDGE_LOOP ( 'NONE', ( #13194, #27657 ) ) ;
#12092=CARTESIAN_POINT ( 'NONE',  ( -0.3065394984451263460, 0.3644188802919184900, 0.1212655228870160168 ) ) ;
#12098=VECTOR ( 'NONE', #776, 39.37007874015748143 ) ;
#12104=CARTESIAN_POINT ( 'NONE',  ( 0.0006615832606325197825, 0.6212594902576319411, 0.09685039370078740717 ) ) ;
#12121=FACE_BOUND ( 'NONE', #1617, .T. ) ;
#12148=EDGE_LOOP ( 'NONE', ( #22079, #6928, #13642, #27, #4314, #15946 ) ) ;
#12155=DIRECTION ( 'NONE',  ( 1.000000000000000000, 0.000000000000000000, 0.000000000000000000 ) ) ;
#12160=CARTESIAN_POINT ( 'NONE',  ( -0.1710938124795999826, -0.4706537664821763833, 0.2574827755769819038 ) ) ;
#12162=CARTESIAN_POINT ( 'NONE',  ( -0.6478824768902187170, 0.1135474080053010398, 0.2081850588238823851 ) ) ;
#12163=EDGE_LOOP ( 'NONE', ( #14445, #21411, #9961, #21902 ) ) ;
#12171=ORIENTED_EDGE ( 'NONE', *, *, #26613, .F. ) ;
#12175=ORIENTED_EDGE ( 'NONE', *, *, #13139, .F. ) ;
#12176=CARTESIAN_POINT ( 'NONE',  ( -0.1918813796216842782, -0.5271897577243779276, 0.1771653543307086520 ) ) ;
#12208=B_SPLINE_CURVE_WITH_KNOTS ( 'NONE', 3,
 ( #1691, #23606, #25427, #14729 ),
 .UNSPECIFIED., .F., .F.,
 ( 4, 4 ),
 ( 0.9046454396443728285, 0.9061502038671860326 ),
 .UNSPECIFIED. ) ;
#12218=ORIENTED_EDGE ( 'NONE', *, *, #13203, .T. ) ;
#12219=CARTESIAN_POINT ( 'NONE',  ( 0.3990005999895503419, 0.4761957181735173017, 0.09684874924366436433 ) ) ;
#12254=ORIENTED_EDGE ( 'NONE', *, *, #24754, .F. ) ;
#12255=CARTESIAN_POINT ( 'NONE',  ( 0.1669561253490893793, -0.4569961989603250618, 0.1075369453269351266 ) ) ;
#12270=CARTESIAN_POINT ( 'NONE',  ( 0.2120693917185543231, -0.5839438448129543602, 0.09684874924366436433 ) ) ;
#12277=CARTESIAN_POINT ( 'NONE',  ( -0.3214446924536846772, 0.3840069416942866742, 0.2574803149606298969 ) ) ;
#12279=DIRECTION ( 'NONE',  ( 0.000000000000000000, 1.000000000000000000, 0.000000000000000000 ) ) ;
#12282=CIRCLE ( 'NONE', #5983, 0.7165354330708662012 ) ;
#12285=CARTESIAN_POINT ( 'NONE',  ( 0.2128972891168984249, -0.5836425148029299459, 0.2574819594177527593 ) ) ;
#12287=EDGE_CURVE ( 'NONE', #22576, #21648, #15112, .T. ) ;
#12289=ORIENTED_EDGE ( 'NONE', *, *, #14410, .F. ) ;
#12329=EDGE_LOOP ( 'NONE', ( #1441, #11281 ) ) ;
#12338=ORIENTED_EDGE ( 'NONE', *, *, #22297, .T. ) ;
#12352=CIRCLE ( 'NONE', #1528, 0.1003956692913385990 ) ;
#12384=FACE_OUTER_BOUND ( 'NONE', #21091, .T. ) ;
#12392=CARTESIAN_POINT ( 'NONE',  ( -0.4688657571743830577, 0.08326155277092069096, 0.1212655228864951557 ) ) ;
#12396=CARTESIAN_POINT ( 'NONE',  ( -0.2256062985779239694, -0.6178563876543621269, 0.2081850588299369031 ) ) ;
#12400=ORIENTED_EDGE ( 'NONE', *, *, #19654, .F. ) ;
#12401=CARTESIAN_POINT ( 'NONE',  ( 0.1634143070181317270, -0.4472844159275946030, 0.1212655228078316633 ) ) ;
#12404=CARTESIAN_POINT ( 'NONE',  ( -0.4256740239330940589, 0.5062356173688730143, 0.1616495878803643205 ) ) ;
#12410=CIRCLE ( 'NONE', #22318, 0.5007874015748031704 ) ;
#12450=EDGE_CURVE ( 'NONE', #13715, #24919, #19906, .T. ) ;
#12452=CARTESIAN_POINT ( 'NONE',  ( 0.4537304931026562849, 0.07942646906837143306, 0.1771653543307087630 ) ) ;
#12456=ORIENTED_EDGE ( 'NONE', *, *, #6586, .T. ) ;
#12463=DIRECTION ( 'NONE',  ( -0.9396926207859083169, -0.3420201433256692125, 0.000000000000000000 ) ) ;
#12466=AXIS2_PLACEMENT_3D ( 'NONE', #24436, #19935, #590 ) ;
#12469=AXIS2_PLACEMENT_3D ( 'NONE', #4984, #7115, #14037 ) ;
#12478=DIRECTION ( 'NONE',  ( 0.000000000000000000, 1.000000000000000000, 0.000000000000000000 ) ) ;
#12484=CARTESIAN_POINT ( 'NONE',  ( -0.2120693917185216271, -0.5839438448129662396, 0.2574819594177527593 ) ) ;
#12490=CARTESIAN_POINT ( 'NONE',  ( 0.000000000000000000, 0.000000000000000000, 0.1771653543307086520 ) ) ;
#12504=CARTESIAN_POINT ( 'NONE',  ( -0.3214446924536846772, 0.3840069416942866742, 0.09685039370078740717 ) ) ;
#12505=ORIENTED_EDGE ( 'NONE', *, *, #8211, .F. ) ;
#12509=CARTESIAN_POINT ( 'NONE',  ( 0.2131049448084480213, -0.5835666837866708700, 0.2574803149606298969 ) ) ;
#12516=DIRECTION ( 'NONE',  ( 1.000000000000000000, 0.000000000000000000, 0.000000000000000000 ) ) ;
#12522=CARTESIAN_POINT ( 'NONE',  ( 0.0001974756197918694275, 0.5007874015748031704, 0.2574827755769819038 ) ) ;
#12536=EDGE_LOOP ( 'NONE', ( #26095, #15084 ) ) ;
#12563=ORIENTED_EDGE ( 'NONE', *, *, #26186, .F. ) ;
#12571=AXIS2_PLACEMENT_3D ( 'NONE', #4685, #471, #8658 ) ;
#12576=EDGE_CURVE ( 'NONE', #8924, #26710, #5471, .T. ) ;
#12581=CYLINDRICAL_SURFACE ( 'NONE', #11112, 0.7283464566929134243 ) ;
#12594=ORIENTED_EDGE ( 'NONE', *, *, #14264, .F. ) ;
#12599=LINE ( 'NONE', #12871, #7606 ) ;
#12607=EDGE_CURVE ( 'NONE', #11359, #9393, #14059, .T. ) ;
#12622=DIRECTION ( 'NONE',  ( 0.000000000000000000, -1.000000000000000000, 0.000000000000000000 ) ) ;
#12624=LINE ( 'NONE', #1885, #1423 ) ;
#12625=ORIENTED_EDGE ( 'NONE', *, *, #19218, .F. ) ;
#12633=DIRECTION ( 'NONE',  ( 0.000000000000000000, 0.000000000000000000, -1.000000000000000000 ) ) ;
#12635=VERTEX_POINT ( 'NONE', #13056 ) ;
#12638=CARTESIAN_POINT ( 'NONE',  ( -0.3122922550266335473, 0.3730863453124460549, 0.1075369453635828670 ) ) ;
#12678=CARTESIAN_POINT ( 'NONE',  ( -0.2982299571022201667, 0.3545282230887890074, 0.2048502514545687270 ) ) ;
#12681=ORIENTED_EDGE ( 'NONE', *, *, #6802, .F. ) ;
#12686=EDGE_LOOP ( 'NONE', ( #10168, #16375, #6960, #21128 ) ) ;
#12688=CIRCLE ( 'NONE', #13147, 0.4606299212598425341 ) ;
#12696=DIRECTION ( 'NONE',  ( 0.000000000000000000, 0.000000000000000000, 1.000000000000000000 ) ) ;
#12699=TOROIDAL_SURFACE ( 'NONE', #8646, 0.4055118110236220486, 0.01181102362204724393 ) ;
#12716=VERTEX_POINT ( 'NONE', #900 ) ;
#12717=ADVANCED_FACE ( 'NONE', ( #3130, #9487 ), #5412, .T. ) ;
#12721=CARTESIAN_POINT ( 'NONE',  ( -0.4690668203718997287, 0.08212126673591825521, 0.2330651857806316507 ) ) ;
#12757=CARTESIAN_POINT ( 'NONE',  ( 0.4133615125891543784, 0.4936731914948853661, 0.2359405056213505492 ) ) ;
#12762=AXIS2_PLACEMENT_3D ( 'NONE', #13761, #3151, #18105 ) ;
#12778=CARTESIAN_POINT ( 'NONE',  ( 0.4009292313364363758, -0.2321359940641732067, 0.2048502514564785326 ) ) ;
#12787=TOROIDAL_SURFACE ( 'NONE', #7811, 0.5610236220472440971, 0.1003937007874015908 ) ;
#12789=CARTESIAN_POINT ( 'NONE',  ( -0.5692936381918457522, -0.3294684677439395637, 0.2081850588301124849 ) ) ;
#12801=CLOSED_SHELL ( 'NONE', ( #9180, #580, #3832, #17393, #4276, #17492, #21556, #16210, #27630, #10037, #300, #21214, #20500, #23651, #26828, #19163, #5681, #18345, #19845, #7631, #27378, #8314, #1285, #1784, #8141, #17048, #13753, #15611, #16856, #13032, #17129, #27324, #22010, #27462, #16373, #10488, #13645, #4920, #4749, #3957, #26907, #63, #26730, #11974, #10926, #26307, #7263, #1026, #6579, #7222, #3576, #14335, #16992, #23014, #2675, #15242, #5581, #7446, #344, #12717, #19871, #1594, #16626, #25631, #4223, #10939, #595, #10363, #24500, #12000, #16144, #8338 ) ) ;
#12816=VERTEX_POINT ( 'NONE', #23333 ) ;
#12841=DIRECTION ( 'NONE',  ( -0.9848077530122077983, 0.1736481776669313304, 0.000000000000000000 ) ) ;
#12846=VERTEX_POINT ( 'NONE', #10301 ) ;
#12858=CARTESIAN_POINT ( 'NONE',  ( -0.4337933494688747671, -0.2502226818840338485, 0.09684793308443542803 ) ) ;
#12871=CARTESIAN_POINT ( 'NONE',  ( -8.919671568592927398E-17, -0.7283464566929134243, 0.1771653543307086520 ) ) ;
#12879=B_SPLINE_CURVE_WITH_KNOTS ( 'NONE', 3,
 ( #8458, #10569, #10855, #8598, #10286, #18902 ),
 .UNSPECIFIED., .F., .F.,
 ( 4, 2, 4 ),
 ( 0.5000000000000000000, 0.7500000000000000000, 1.000000000000000000 ),
 .UNSPECIFIED. ) ;
#12883=CIRCLE ( 'NONE', #21929, 0.6212598425196850238 ) ;
#12884=CARTESIAN_POINT ( 'NONE',  ( 0.1580799066051618851, -0.4326553680327471785, 0.1771653543307085410 ) ) ;
#12894=CARTESIAN_POINT ( 'NONE',  ( -0.4792483803599256187, 0.08390985360213192024, 0.1075369453628696598 ) ) ;
#12896=ORIENTED_EDGE ( 'NONE', *, *, #27181, .T. ) ;
#12914=DIRECTION ( 'NONE',  ( 0.000000000000000000, 0.000000000000000000, 1.000000000000000000 ) ) ;
#12919=VERTEX_POINT ( 'NONE', #16765 ) ;
#12921=CARTESIAN_POINT ( 'NONE',  ( -0.5376957092749645728, -0.3112026930392425284, 0.09685039370078740717 ) ) ;
#12931=DIRECTION ( 'NONE',  ( 0.000000000000000000, 0.000000000000000000, -1.000000000000000000 ) ) ;
#12954=DIRECTION ( 'NONE',  ( 1.000000000000000000, 0.000000000000000000, 0.000000000000000000 ) ) ;
#12958=LINE ( 'NONE', #6068, #15639 ) ;
#12962=ORIENTED_EDGE ( 'NONE', *, *, #3694, .F. ) ;
#12988=CARTESIAN_POINT ( 'NONE',  ( -0.1669561253486535057, -0.4569961989591353468, 0.1075369453278852555 ) ) ;
#12997=FACE_OUTER_BOUND ( 'NONE', #4601, .T. ) ;
#13004=CARTESIAN_POINT ( 'NONE',  ( 0.1570092758121679200, -0.4330450457732857861, 0.1771653543307087630 ) ) ;
#13007=CARTESIAN_POINT ( 'NONE',  ( 0.5572789388074469441, -0.3225230913461603066, 0.1183902030391640881 ) ) ;
#13019=ORIENTED_EDGE ( 'NONE', *, *, #6413, .F. ) ;
#13020=ORIENTED_EDGE ( 'NONE', *, *, #22197, .T. ) ;
#13028=ORIENTED_EDGE ( 'NONE', *, *, #17207, .T. ) ;
#13029=FACE_OUTER_BOUND ( 'NONE', #3523, .T. ) ;
#13032=ADVANCED_FACE ( 'NONE', ( #12384 ), #2943, .T. ) ;
#13042=DIRECTION ( 'NONE',  ( 0.000000000000000000, 1.000000000000000000, 0.000000000000000000 ) ) ;
#13051=DIRECTION ( 'NONE',  ( 0.000000000000000000, 1.000000000000000000, 0.000000000000000000 ) ) ;
#13056=CARTESIAN_POINT ( 'NONE',  ( 0.3223547283257516272, 0.3832433309296771617, 0.09685039370078740717 ) ) ;
#13060=DIRECTION ( 'NONE',  ( 0.000000000000000000, 0.000000000000000000, -1.000000000000000000 ) ) ;
#13061=CARTESIAN_POINT ( 'NONE',  ( 0.3995066426835866547, 0.4757712504659488140, 0.2574827755769819038 ) ) ;
#13073=EDGE_CURVE ( 'NONE', #15131, #4007, #12282, .T. ) ;
#13077=CARTESIAN_POINT ( 'NONE',  ( 0.3065394984556240598, 0.3644188803044271507, 0.1212655228622371850 ) ) ;
#13083=CIRCLE ( 'NONE', #10374, 0.4606299212598425341 ) ;
#13090=AXIS2_PLACEMENT_3D ( 'NONE', #11459, #9465, #731 ) ;
#13099=ORIENTED_EDGE ( 'NONE', *, *, #5501, .F. ) ;
#13109=CARTESIAN_POINT ( 'NONE',  ( 0.5376957092749897749, -0.3112026930391976753, 0.2574803149606298969 ) ) ;
#13113=CARTESIAN_POINT ( 'NONE',  ( 0.000000000000000000, 0.000000000000000000, 0.1771653543307086520 ) ) ;
#13120=AXIS2_PLACEMENT_3D ( 'NONE', #24767, #9654, #25190 ) ;
#13130=VERTEX_POINT ( 'NONE', #21705 ) ;
#13134=EDGE_CURVE ( 'NONE', #5560, #20533, #19505, .T. ) ;
#13139=EDGE_CURVE ( 'NONE', #15868, #20920, #13377, .T. ) ;
#13142=CARTESIAN_POINT ( 'NONE',  ( 0.5692936381913840105, -0.3294684677436600095, 0.1461456498297685480 ) ) ;
#13147=AXIS2_PLACEMENT_3D ( 'NONE', #6602, #139, #19310 ) ;
#13166=CARTESIAN_POINT ( 'NONE',  ( -0.4333973147258542991, -0.2509079296564011852, 0.2574803149606298969 ) ) ;
#13175=DIRECTION ( 'NONE',  ( 0.000000000000000000, 0.000000000000000000, 1.000000000000000000 ) ) ;
#13185=CARTESIAN_POINT ( 'NONE',  ( -0.0006737210091386627636, 0.6438792636747241449, 0.2359405056217873942 ) ) ;
#13188=VERTEX_POINT ( 'NONE', #5139 ) ;
#13194=ORIENTED_EDGE ( 'NONE', *, *, #18637, .F. ) ;
#13198=FACE_BOUND ( 'NONE', #9586, .T. ) ;
#13203=EDGE_CURVE ( 'NONE', #16353, #20701, #24020, .T. ) ;
#13204=B_SPLINE_CURVE_WITH_KNOTS ( 'NONE', 3,
 ( #1282, #7782, #18490, #5662, #1555, #27137 ),
 .UNSPECIFIED., .F., .F.,
 ( 4, 2, 4 ),
 ( 0.5000000000000000000, 0.7500000000000000000, 1.000000000000000000 ),
 .UNSPECIFIED. ) ;
#13207=DIRECTION ( 'NONE',  ( -0.6427876096865392519, 0.7660444431189780135, 0.000000000000000000 ) ) ;
#13210=CARTESIAN_POINT ( 'NONE',  ( -0.2118615749922956593, -0.5840192333899354438, 0.09685039370078740717 ) ) ;
#13214=ORIENTED_EDGE ( 'NONE', *, *, #3902, .T. ) ;
#13215=FACE_OUTER_BOUND ( 'NONE', #9355, .T. ) ;
#13218=VERTEX_POINT ( 'NONE', #26473 ) ;
#13221=VERTEX_POINT ( 'NONE', #13210 ) ;
#13235=VERTEX_POINT ( 'NONE', #17850 ) ;
#13265=( CONVERSION_BASED_UNIT ( 'INCH', #4638 ) LENGTH_UNIT ( ) NAMED_UNIT ( #6740 ) ) ;
#13279=DIRECTION ( 'NONE',  ( 0.000000000000000000, 0.000000000000000000, 1.000000000000000000 ) ) ;
#13283=CARTESIAN_POINT ( 'NONE',  ( 0.000000000000000000, 0.000000000000000000, 0.2574803149606298969 ) ) ;
#13284=VECTOR ( 'NONE', #18917, 39.37007874015748143 ) ;
#13295=CARTESIAN_POINT ( 'NONE',  ( 0.000000000000000000, 0.000000000000000000, 0.1771653543307086520 ) ) ;
#13296=ORIENTED_EDGE ( 'NONE', *, *, #17460, .F. ) ;
#13298=ORIENTED_EDGE ( 'NONE', *, *, #26914, .T. ) ;
#13327=CIRCLE ( 'NONE', #22339, 0.1003956692913385851 ) ;
#13342=CARTESIAN_POINT ( 'NONE',  ( 0.0005855335178282750032, 0.4865383137623722209, 0.1075369453635709044 ) ) ;
#13346=TOROIDAL_SURFACE ( 'NONE', #25981, 0.5610236220472440971, 0.1003937007874015908 ) ;
#13375=ORIENTED_EDGE ( 'NONE', *, *, #8711, .T. ) ;
#13377=B_SPLINE_CURVE_WITH_KNOTS ( 'NONE', 3,
 ( #4468, #10680, #17321, #25939, #23696, #6592 ),
 .UNSPECIFIED., .F., .F.,
 ( 4, 2, 4 ),
 ( 0.9359046326925629655, 0.9375808709372039917, 0.9392571091818440188 ),
 .UNSPECIFIED. ) ;
#13411=CARTESIAN_POINT ( 'NONE',  ( -0.3992017438595018564, -0.2298214351608254269, 0.1771653543307087630 ) ) ;
#13430=ORIENTED_EDGE ( 'NONE', *, *, #8614, .F. ) ;
#13435=CARTESIAN_POINT ( 'NONE',  ( -0.6117448998508523417, 0.1083144418130960601, 0.09684874924366436433 ) ) ;
#13437=DIRECTION ( 'NONE',  ( 0.000000000000000000, 0.000000000000000000, 1.000000000000000000 ) ) ;
#13449=ORIENTED_EDGE ( 'NONE', *, *, #15648, .T. ) ;
#13452=CARTESIAN_POINT ( 'NONE',  ( -0.4688657571743239938, 0.08326155277091105977, 0.2330651857748314848 ) ) ;
#13455=AXIS2_PLACEMENT_3D ( 'NONE', #12490, #21108, #10639 ) ;
#13462=CYLINDRICAL_SURFACE ( 'NONE', #18121, 0.7283464566929134243 ) ;
#13475=AXIS2_PLACEMENT_3D ( 'NONE', #2442, #23933, #6189 ) ;
#13477=CARTESIAN_POINT ( 'NONE',  ( 0.3223547283257516272, 0.3832433309296771617, 0.09685039370078740717 ) ) ;
#13488=SHAPE_DEFINITION_REPRESENTATION ( #16330, #1615 ) ;
#13493=ORIENTED_EDGE ( 'NONE', *, *, #4541, .F. ) ;
#13512=EDGE_CURVE ( 'NONE', #15905, #23049, #14326, .T. ) ;
#13521=CARTESIAN_POINT ( 'NONE',  ( -0.3990005999895503419, 0.4761957181735173017, 0.09684874924366436433 ) ) ;
#13523=CARTESIAN_POINT ( 'NONE',  ( -0.3986320731132244610, -0.2308081338369635804, 0.1771653543307087630 ) ) ;
#13527=CARTESIAN_POINT ( 'NONE',  ( 0.4009292313359112958, -0.2321359940638691999, 0.1494804572070806692 ) ) ;
#13528=VERTEX_POINT ( 'NONE', #8501 ) ;
#13536=DIRECTION ( 'NONE',  ( 0.000000000000000000, 0.000000000000000000, 1.000000000000000000 ) ) ;
#13547=CARTESIAN_POINT ( 'NONE',  ( 0.5525004126151165096, 0.09742072959660433296, 0.2775610236220472093 ) ) ;
#13572=CYLINDRICAL_SURFACE ( 'NONE', #13090, 0.5007874015748031704 ) ;
#13576=CARTESIAN_POINT ( 'NONE',  ( 0.000000000000000000, 0.000000000000000000, 0.1771653543307086520 ) ) ;
#13579=FACE_BOUND ( 'NONE', #2781, .T. ) ;
#13599=CARTESIAN_POINT ( 'NONE',  ( 0.4078284417476525925, 0.4849914877851788098, 0.1061598535658143105 ) ) ;
#13606=CARTESIAN_POINT ( 'NONE',  ( 0.3988311005572732215, 0.4763376377695315300, 0.2574803149606298969 ) ) ;
#13616=DIRECTION ( 'NONE',  ( 0.000000000000000000, 0.000000000000000000, 1.000000000000000000 ) ) ;
#13617=B_SPLINE_CURVE_WITH_KNOTS ( 'NONE', 3,
 ( #24881, #9330, #887, #22765, #13725, #18509 ),
 .UNSPECIFIED., .F., .F.,
 ( 4, 2, 4 ),
 ( 0.9031406754215589583, 0.9046454396443720514, 0.9061502038671860326 ),
 .UNSPECIFIED. ) ;
#13622=CARTESIAN_POINT ( 'NONE',  ( 0.6339803004448225643, 0.1124719464477440256, 0.2359405056222393382 ) ) ;
#13634=CIRCLE ( 'NONE', #14092, 0.7283464566929134243 ) ;
#13642=ORIENTED_EDGE ( 'NONE', *, *, #10461, .F. ) ;
#13645=ADVANCED_FACE ( 'NONE', ( #15299 ), #12787, .F. ) ;
#13651=DIRECTION ( 'NONE',  ( -0.3420201433256691570, -0.9396926207859082059, 0.000000000000000000 ) ) ;
#13664=B_SPLINE_CURVE_WITH_KNOTS ( 'NONE', 3,
 ( #24454, #17822, #747, #9336, #26575, #5105 ),
 .UNSPECIFIED., .F., .F.,
 ( 4, 2, 4 ),
 ( 0.9359046326925619663, 0.9375808709372029925, 0.9392571091818430196 ),
 .UNSPECIFIED. ) ;
#13680=ORIENTED_EDGE ( 'NONE', *, *, #10914, .F. ) ;
#13686=CARTESIAN_POINT ( 'NONE',  ( 0.000000000000000000, 0.000000000000000000, 0.09685039370078740717 ) ) ;
#13713=AXIS2_PLACEMENT_3D ( 'NONE', #13295, #6947, #21919 ) ;
#13715=VERTEX_POINT ( 'NONE', #1401 ) ;
#13716=CARTESIAN_POINT ( 'NONE',  ( -0.2161007281678285485, -0.5956855348332250610, 0.1061598535668862309 ) ) ;
#13725=CARTESIAN_POINT ( 'NONE',  ( -0.4932478747986535628, 0.08657132889677658649, 0.2574819596263889787 ) ) ;
#13736=DIRECTION ( 'NONE',  ( 0.5000000000000002220, 0.8660254037844383745, 0.000000000000000000 ) ) ;
#13751=CARTESIAN_POINT ( 'NONE',  ( 0.5731455175600789209, -0.3301167833454101141, 0.1926811207747196886 ) ) ;
#13753=ADVANCED_FACE ( 'NONE', ( #22738 ), #7345, .F. ) ;
#13761=CARTESIAN_POINT ( 'NONE',  ( 0.000000000000000000, 0.000000000000000000, 0.3425196850393700809 ) ) ;
#13775=DIRECTION ( 'NONE',  ( 0.000000000000000000, 1.000000000000000000, 0.000000000000000000 ) ) ;
#13811=CARTESIAN_POINT ( 'NONE',  ( -0.3996755081322992398, 0.4756294029998582307, 0.09684874924366436433 ) ) ;
#13818=AXIS2_PLACEMENT_3D ( 'NONE', #2717, #22647, #20103 ) ;
#13832=PRODUCT_DEFINITION_FORMATION_WITH_SPECIFIED_SOURCE ( 'ANY', '', #21073, .NOT_KNOWN. ) ;
#13834=CARTESIAN_POINT ( 'NONE',  ( 0.4931450244001936989, 0.08715529520342342462, 0.2574827755769819038 ) ) ;
#13836=DIRECTION ( 'NONE',  ( 0.000000000000000000, 0.000000000000000000, 1.000000000000000000 ) ) ;
#13867=ORIENTED_EDGE ( 'NONE', *, *, #20703, .T. ) ;
#13884=CARTESIAN_POINT ( 'NONE',  ( 0.3214446924536846772, 0.3840069416942866742, 0.2574803149606298969 ) ) ;
#13902=DIRECTION ( 'NONE',  ( -1.000000000000000000, 0.000000000000000000, 0.000000000000000000 ) ) ;
#13907=VERTEX_POINT ( 'NONE', #23464 ) ;
#13919=ORIENTED_EDGE ( 'NONE', *, *, #4412, .F. ) ;
#13945=CARTESIAN_POINT ( 'NONE',  ( 1.456051859513969730E-17, 0.5007874015748032814, 0.2574827755769819038 ) ) ;
#13950=CARTESIAN_POINT ( 'NONE',  ( 0.4561454261137161126, 0.08101060747726872291, 0.1494804571740294685 ) ) ;
#13954=ORIENTED_EDGE ( 'NONE', *, *, #3428, .T. ) ;
#13956=CARTESIAN_POINT ( 'NONE',  ( -0.4561454261040128744, 0.08101060747557438380, 0.1494804572088045402 ) ) ;
#13968=EDGE_CURVE ( 'NONE', #26393, #10201, #27701, .T. ) ;
#13974=EDGE_CURVE ( 'NONE', #13528, #25113, #210, .T. ) ;
#13993=CARTESIAN_POINT ( 'NONE',  ( 0.2126900928101220500, -0.5837180524351338606, 0.2574827755769819038 ) ) ;
#14010=ORIENTED_EDGE ( 'NONE', *, *, #18061, .T. ) ;
#14032=CARTESIAN_POINT ( 'NONE',  ( 0.4233199042375110910, 0.5034331896104039528, 0.2081850588264056445 ) ) ;
#14033=ORIENTED_EDGE ( 'NONE', *, *, #3309, .F. ) ;
#14037=DIRECTION ( 'NONE',  ( 0.9396926207859082059, 0.3420201433256690460, 0.000000000000000000 ) ) ;
#14059=CIRCLE ( 'NONE', #21268, 0.1003956692913385990 ) ;
#14062=CARTESIAN_POINT ( 'NONE',  ( 0.000000000000000000, 0.000000000000000000, 0.2574803149606298969 ) ) ;
#14064=VERTEX_POINT ( 'NONE', #19473 ) ;
#14078=CARTESIAN_POINT ( 'NONE',  ( -0.2965233727166469713, 0.3524965443697188894, 0.1639447408842210907 ) ) ;
#14079=CARTESIAN_POINT ( 'NONE',  ( 0.000000000000000000, 0.000000000000000000, 0.01181102362204724393 ) ) ;
#14086=CARTESIAN_POINT ( 'NONE',  ( 0.5381367953592983699, -0.3104394140547701020, 0.2574827755769819038 ) ) ;
#14087=AXIS2_PLACEMENT_3D ( 'NONE', #10980, #2089, #12954 ) ;
#14090=CARTESIAN_POINT ( 'NONE',  ( -0.5376957092749645728, -0.3112026930392425284, 0.09685039370078740717 ) ) ;
#14092=AXIS2_PLACEMENT_3D ( 'NONE', #5067, #13836, #15683 ) ;
#14098=FACE_OUTER_BOUND ( 'NONE', #11634, .T. ) ;
#14105=CARTESIAN_POINT ( 'NONE',  ( 0.000000000000000000, 0.5610236220472440971, -3.341531889763779686E-17 ) ) ;
#14112=CARTESIAN_POINT ( 'NONE',  ( 0.4337933494688747671, -0.2502226818840338485, 0.09684793308443523374 ) ) ;
#14120=CARTESIAN_POINT ( 'NONE',  ( 0.4932136069632150344, 0.08676634416061969335, 0.2574827755769819038 ) ) ;
#14142=EDGE_CURVE ( 'NONE', #23041, #13221, #16677, .T. ) ;
#14145=EDGE_LOOP ( 'NONE', ( #16259, #8323, #18569, #7965, #14197 ) ) ;
#14152=VERTEX_POINT ( 'NONE', #24128 ) ;
#14159=CARTESIAN_POINT ( 'NONE',  ( -0.1707210962531915677, -0.4707890492249701131, 0.2574803149606298969 ) ) ;
#14178=EDGE_CURVE ( 'NONE', #13235, #8311, #22254, .T. ) ;
#14182=ORIENTED_EDGE ( 'NONE', *, *, #2987, .F. ) ;
#14184=LINE ( 'NONE', #11765, #26006 ) ;
#14192=CARTESIAN_POINT ( 'NONE',  ( 0.5731455175603656915, -0.3301167833455752043, 0.1616495878888389581 ) ) ;
#14197=ORIENTED_EDGE ( 'NONE', *, *, #23397, .T. ) ;
#14199=EDGE_LOOP ( 'NONE', ( #16880, #22022, #2789, #21576 ) ) ;
#14211=ORIENTED_EDGE ( 'NONE', *, *, #8042, .T. ) ;
#14228=VERTEX_POINT ( 'NONE', #818 ) ;
#14234=AXIS2_PLACEMENT_3D ( 'NONE', #7281, #12914, #21539 ) ;
#14244=CARTESIAN_POINT ( 'NONE',  ( 0.0006737210091407729463, 0.6438792636759185228, 0.1183902030411692757 ) ) ;
#14253=DIRECTION ( 'NONE',  ( 0.000000000000000000, 0.000000000000000000, 1.000000000000000000 ) ) ;
#14260=CARTESIAN_POINT ( 'NONE',  ( 0.2195865873852730354, -0.6052790189071695082, 0.1183902030380611092 ) ) ;
#14264=EDGE_CURVE ( 'NONE', #13528, #17285, #20721, .T. ) ;
#14268=ORIENTED_EDGE ( 'NONE', *, *, #10320, .F. ) ;
#14274=DIRECTION ( 'NONE',  ( 1.000000000000000000, 0.000000000000000000, 0.000000000000000000 ) ) ;
#14276=EDGE_LOOP ( 'NONE', ( #7328, #14211 ) ) ;
#14286=ORIENTED_EDGE ( 'NONE', *, *, #26922, .T. ) ;
#14289=CARTESIAN_POINT ( 'NONE',  ( -0.3222028160008074682, 0.3833711078595924970, 0.09684874903502814492 ) ) ;
#14307=DIRECTION ( 'NONE',  ( 0.000000000000000000, 0.000000000000000000, 1.000000000000000000 ) ) ;
#14310=CARTESIAN_POINT ( 'NONE',  ( -0.3937007874015748254, 4.893765752498281459E-17, 0.01181102362204724393 ) ) ;
#14319=ORIENTED_EDGE ( 'NONE', *, *, #21493, .T. ) ;
#14326=B_SPLINE_CURVE_WITH_KNOTS ( 'NONE', 3,
 ( #21221, #1862, #27864, #10469, #19086, #23207 ),
 .UNSPECIFIED., .F., .F.,
 ( 4, 2, 4 ),
 ( 0.5000000000000000000, 0.7500000000000000000, 1.000000000000000000 ),
 .UNSPECIFIED. ) ;
#14328=CARTESIAN_POINT ( 'NONE',  ( 0.000000000000000000, 0.000000000000000000, 0.1771653543307086520 ) ) ;
#14335=ADVANCED_FACE ( 'NONE', ( #26505 ), #26768, .F. ) ;
#14353=SURFACE_STYLE_FILL_AREA ( #18705 ) ;
#14367=B_SPLINE_CURVE_WITH_KNOTS ( 'NONE', 3,
 ( #12504, #12638, #16890, #17026, #27765, #25073 ),
 .UNSPECIFIED., .F., .F.,
 ( 4, 2, 4 ),
 ( 0.000000000000000000, 0.2500000000000000000, 0.5000000000000000000 ),
 .UNSPECIFIED. ) ;
#14369=VERTEX_POINT ( 'NONE', #21294 ) ;
#14386=EDGE_CURVE ( 'NONE', #10869, #6124, #18292, .T. ) ;
#14387=CARTESIAN_POINT ( 'NONE',  ( -0.0005855335178275720065, 0.4865383137617886322, 0.1075369453640087208 ) ) ;
#14398=EDGE_LOOP ( 'NONE', ( #26277, #27213, #11239, #466, #14441 ) ) ;
#14410=EDGE_CURVE ( 'NONE', #21729, #22901, #20469, .T. ) ;
#14416=CARTESIAN_POINT ( 'NONE',  ( 0.2122766679520240174, -0.5838685267775873822, 0.09684793308443542803 ) ) ;
#14421=DIRECTION ( 'NONE',  ( 0.000000000000000000, 1.000000000000000000, 0.000000000000000000 ) ) ;
#14429=CARTESIAN_POINT ( 'NONE',  ( 0.5525004126151165096, 0.09742072959660433296, 0.1771653543307086520 ) ) ;
#14441=ORIENTED_EDGE ( 'NONE', *, *, #19919, .F. ) ;
#14445=ORIENTED_EDGE ( 'NONE', *, *, #17628, .T. ) ;
#14452=CARTESIAN_POINT ( 'NONE',  ( -0.6119360453657125554, 0.1072290460171901605, 0.09685039370078740717 ) ) ;
#14477=AXIS2_PLACEMENT_3D ( 'NONE', #2637, #24387, #9398 ) ;
#14483=ORIENTED_EDGE ( 'NONE', *, *, #12450, .F. ) ;
#14488=ORIENTED_EDGE ( 'NONE', *, *, #26400, .T. ) ;
#14493=B_SPLINE_CURVE_WITH_KNOTS ( 'NONE', 3,
 ( #27487, #27769, #12778, #3888, #8274, #15195 ),
 .UNSPECIFIED., .F., .F.,
 ( 4, 2, 4 ),
 ( 0.5000000000000000000, 0.7500000000000000000, 1.000000000000000000 ),
 .UNSPECIFIED. ) ;
#14509=EDGE_CURVE ( 'NONE', #11779, #5913, #6834, .T. ) ;
#14545=EDGE_CURVE ( 'NONE', #15551, #17891, #2159, .T. ) ;
#14579=DIRECTION ( 'NONE',  ( -0.4999999999999997780, 0.8660254037844388186, 0.000000000000000000 ) ) ;
#14597=CARTESIAN_POINT ( 'NONE',  ( 0.1707210962531913734, -0.4707890492249701131, 0.09685039370078740717 ) ) ;
#14599=CARTESIAN_POINT ( 'NONE',  ( -0.1658556822965989719, -0.4573967274740618483, 0.1075369453282564308 ) ) ;
#14609=CARTESIAN_POINT ( 'NONE',  ( 0.1918813796216842782, -0.5271897577243779276, 0.1771653543307086520 ) ) ;
#14628=ORIENTED_EDGE ( 'NONE', *, *, #13073, .T. ) ;
#14635=ORIENTED_EDGE ( 'NONE', *, *, #13203, .F. ) ;
#14644=EDGE_CURVE ( 'NONE', #12919, #6711, #20935, .T. ) ;
#14646=VERTEX_POINT ( 'NONE', #14310 ) ;
#14651=( CONVERSION_BASED_UNIT ( 'INCH', #16739 ) LENGTH_UNIT ( ) NAMED_UNIT ( #7979 ) ) ;
#14654=AXIS2_PLACEMENT_3D ( 'NONE', #15300, #12633, #1894 ) ;
#14658=ORIENTED_EDGE ( 'NONE', *, *, #25561, .T. ) ;
#14659=VERTEX_POINT ( 'NONE', #18660 ) ;
#14673=CARTESIAN_POINT ( 'NONE',  ( 0.4535326485287339282, 0.08054850140356757671, 0.1771653543307084855 ) ) ;
#14675=AXIS2_PLACEMENT_3D ( 'NONE', #14429, #11724, #18200 ) ;
#14677=CARTESIAN_POINT ( 'NONE',  ( 0.0006832381873096096290, 0.6614169699447792761, 0.1926811207755882993 ) ) ;
#14682=ORIENTED_EDGE ( 'NONE', *, *, #14893, .T. ) ;
#14687=CARTESIAN_POINT ( 'NONE',  ( -0.2256062985780004637, -0.6178563876545716260, 0.1461456498321150876 ) ) ;
#14699=ORIENTED_EDGE ( 'NONE', *, *, #26922, .F. ) ;
#14701=EDGE_CURVE ( 'NONE', #5816, #27022, #22774, .T. ) ;
#14708=EDGE_CURVE ( 'NONE', #6078, #3924, #27726, .T. ) ;
#14710=CARTESIAN_POINT ( 'NONE',  ( -0.0005710523241074312757, 0.4632828964890012835, 0.2048502514557469789 ) ) ;
#14713=VERTEX_POINT ( 'NONE', #10186 ) ;
#14719=B_SPLINE_CURVE_WITH_KNOTS ( 'NONE', 3,
 ( #24168, #17793, #20199, #15826, #2952, #22461 ),
 .UNSPECIFIED., .F., .F.,
 ( 4, 2, 4 ),
 ( 0.5000000000000000000, 0.7500000000000000000, 1.000000000000000000 ),
 .UNSPECIFIED. ) ;
#14720=APPLICATION_CONTEXT ( 'automotive_design' ) ;
#14729=CARTESIAN_POINT ( 'NONE',  ( -0.0005939837304750000086, 0.5007870493127504208, 0.2574803149606298969 ) ) ;
#14744=DIRECTION ( 'NONE',  ( 0.000000000000000000, 0.000000000000000000, 1.000000000000000000 ) ) ;
#14747=DIRECTION ( 'NONE',  ( 0.000000000000000000, 0.000000000000000000, 1.000000000000000000 ) ) ;
#14759=ORIENTED_EDGE ( 'NONE', *, *, #8608, .T. ) ;
#14763=TOROIDAL_SURFACE ( 'NONE', #8400, 0.5610236220472440971, 0.1003937007874015908 ) ;
#14770=CARTESIAN_POINT ( 'NONE',  ( -0.1707210962531915677, -0.4707890492249701131, 0.09685039370078740717 ) ) ;
#14820=EDGE_LOOP ( 'NONE', ( #22242, #20673 ) ) ;
#14839=EDGE_LOOP ( 'NONE', ( #7003, #22475, #21716, #10305, #1193, #21265 ) ) ;
#14842=B_SPLINE_CURVE_WITH_KNOTS ( 'NONE', 3,
 ( #27154, #3532, #1429, #10043 ),
 .UNSPECIFIED., .F., .F.,
 ( 4, 4 ),
 ( 0.3000437156586439613, 0.3015484798814578316 ),
 .UNSPECIFIED. ) ;
#14845=CARTESIAN_POINT ( 'NONE',  ( -0.0005696707463066809363, 0.4606295689977896179, 0.1903859677778869663 ) ) ;
#14868=ORIENTED_EDGE ( 'NONE', *, *, #7300, .T. ) ;
#14870=CARTESIAN_POINT ( 'NONE',  ( 0.4931450244001936989, 0.08715529520342342462, 0.09684793308443523374 ) ) ;
#14880=CARTESIAN_POINT ( 'NONE',  ( -0.4563437504967154390, 0.07988585396358348356, 0.2048502514591916679 ) ) ;
#14881=CARTESIAN_POINT ( 'NONE',  ( 0.000000000000000000, 0.000000000000000000, 0.2574803149606298969 ) ) ;
#14885=CARTESIAN_POINT ( 'NONE',  ( -0.1707210962531915677, -0.4707890492249701131, 0.09685039370078740717 ) ) ;
#14893=EDGE_CURVE ( 'NONE', #11904, #19560, #225, .T. ) ;
#14894=CIRCLE ( 'NONE', #10338, 0.1003956692913385573 ) ;
#14895=AXIS2_PLACEMENT_3D ( 'NONE', #4561, #8796, #17414 ) ;
#14904=EDGE_LOOP ( 'NONE', ( #274, #22549, #17838, #512 ) ) ;
#14907=CARTESIAN_POINT ( 'NONE',  ( 0.4068047116062469826, 0.4858504993706820874, 0.1061598535666330306 ) ) ;
#14910=CIRCLE ( 'NONE', #24787, 0.3937007874015748254 ) ;
#14919=CIRCLE ( 'NONE', #4955, 0.3937007874015748254 ) ;
#14935=VERTEX_POINT ( 'NONE', #19930 ) ;
#14943=CARTESIAN_POINT ( 'NONE',  ( 0.4930758245789425009, 0.08754571829529310401, 0.2574803149606298969 ) ) ;
#14950=ORIENTED_EDGE ( 'NONE', *, *, #969, .F. ) ;
#14960=CARTESIAN_POINT ( 'NONE',  ( -0.6512499169102675678, 0.1155267097730827697, 0.1926811207693707451 ) ) ;
#14967=ORIENTED_EDGE ( 'NONE', *, *, #27695, .F. ) ;
#14975=CARTESIAN_POINT ( 'NONE',  ( 0.000000000000000000, 0.000000000000000000, -3.278217716535432842E-17 ) ) ;
#14980=CARTESIAN_POINT ( 'NONE',  ( 0.4216473063920845865, -0.2427620699802750248, 0.2467937632982898366 ) ) ;
#14985=CIRCLE ( 'NONE', #10890, 0.1003956692913385851 ) ;
#14988=FACE_OUTER_BOUND ( 'NONE', #1224, .T. ) ;
#15005=CARTESIAN_POINT ( 'NONE',  ( 0.3214446924536846772, 0.3840069416942866742, 0.2574803149606298969 ) ) ;
#15012=CARTESIAN_POINT ( 'NONE',  ( 0.1658556822975960354, -0.4573967274768249713, 0.1075369453260532765 ) ) ;
#15037=CARTESIAN_POINT ( 'NONE',  ( -0.4932821129636645874, 0.08637579872942342807, 0.09685039370078740717 ) ) ;
#15038=CARTESIAN_POINT ( 'NONE',  ( -0.3995066426835598983, 0.4757712504659716291, 0.2574827755769819038 ) ) ;
#15046=EDGE_CURVE ( 'NONE', #14659, #17723, #3349, .T. ) ;
#15055=ORIENTED_EDGE ( 'NONE', *, *, #27121, .F. ) ;
#15084=ORIENTED_EDGE ( 'NONE', *, *, #588, .T. ) ;
#15085=CARTESIAN_POINT ( 'NONE',  ( 0.000000000000000000, 0.000000000000000000, -3.278217716535432842E-17 ) ) ;
#15094=DIRECTION ( 'NONE',  ( 0.000000000000000000, 1.000000000000000000, 0.000000000000000000 ) ) ;
#15097=CARTESIAN_POINT ( 'NONE',  ( -0.6117062799105453808, 0.1085321106658580781, 0.09685039370078740717 ) ) ;
#15108=CARTESIAN_POINT ( 'NONE',  ( 0.6118978891064172920, 0.1074467966294246069, 0.09684874924366436433 ) ) ;
#15109=ORIENTED_EDGE ( 'NONE', *, *, #8618, .F. ) ;
#15112=B_SPLINE_CURVE_WITH_KNOTS ( 'NONE', 3,
 ( #17192, #17465, #25808, #6456, #23837, #23702 ),
 .UNSPECIFIED., .F., .F.,
 ( 4, 2, 4 ),
 ( 0.000000000000000000, 0.2500000000000000000, 0.5000000000000000000 ),
 .UNSPECIFIED. ) ;
#15131=VERTEX_POINT ( 'NONE', #27264 ) ;
#15133=CARTESIAN_POINT ( 'NONE',  ( 0.1634143070183528834, -0.4472844159282008958, 0.2330651858545649824 ) ) ;
#15135=CARTESIAN_POINT ( 'NONE',  ( -0.1718374205099799101, -0.4703827404237102550, 0.09685039370078740717 ) ) ;
#15150=CARTESIAN_POINT ( 'NONE',  ( 0.1623262587471781815, -0.4476804331129728975, 0.1212655228059691948 ) ) ;
#15152=DIRECTION ( 'NONE',  ( 0.000000000000000000, -1.000000000000000000, 0.000000000000000000 ) ) ;
#15155=B_SPLINE_CURVE_WITH_KNOTS ( 'NONE', 3,
 ( #16996, #23780, #25471, #21653, #10769, #342 ),
 .UNSPECIFIED., .F., .F.,
 ( 4, 2, 4 ),
 ( 0.5000000000000000000, 0.7500000000000000000, 1.000000000000000000 ),
 .UNSPECIFIED. ) ;
#15163=ORIENTED_EDGE ( 'NONE', *, *, #6634, .F. ) ;
#15165=ORIENTED_EDGE ( 'NONE', *, *, #17447, .F. ) ;
#15195=CARTESIAN_POINT ( 'NONE',  ( 0.4333973147258542991, -0.2509079296564015737, 0.2574803149606298969 ) ) ;
#15196=CARTESIAN_POINT ( 'NONE',  ( 0.2268599607409950980, -0.6212949646958005889, 0.1616495878780456474 ) ) ;
#15204=FACE_OUTER_BOUND ( 'NONE', #7614, .T. ) ;
#15205=CARTESIAN_POINT ( 'NONE',  ( -0.4339912984563299436, -0.2498791196563492356, 0.09685039370078740717 ) ) ;
#15229=STYLED_ITEM ( 'NONE', ( #27342 ), #22049 ) ;
#15230=ORIENTED_EDGE ( 'NONE', *, *, #6459, .F. ) ;
#15234=CARTESIAN_POINT ( 'NONE',  ( 0.0006615832606325197825, 0.6212594902576319411, 0.09685039370078740717 ) ) ;
#15242=ADVANCED_FACE ( 'NONE', ( #14988, #1970 ), #6223, .T. ) ;
#15245=EDGE_LOOP ( 'NONE', ( #21196, #19169, #16123, #5999, #10240, #18568 ) ) ;
#15264=EDGE_CURVE ( 'NONE', #24998, #6679, #12208, .T. ) ;
#15272=DIRECTION ( 'NONE',  ( 0.000000000000000000, 0.000000000000000000, -1.000000000000000000 ) ) ;
#15286=DIRECTION ( 'NONE',  ( 0.000000000000000000, 1.000000000000000000, 0.000000000000000000 ) ) ;
#15292=CIRCLE ( 'NONE', #11771, 0.5007874015748031704 ) ;
#15294=CARTESIAN_POINT ( 'NONE',  ( -0.7283464566929135353, 8.919671568592928630E-17, 0.3425196850393700809 ) ) ;
#15299=FACE_OUTER_BOUND ( 'NONE', #5341, .T. ) ;
#15300=CARTESIAN_POINT ( 'NONE',  ( 0.000000000000000000, 0.000000000000000000, 0.3543307086614173040 ) ) ;
#15304=ORIENTED_EDGE ( 'NONE', *, *, #9099, .T. ) ;
#15325=CARTESIAN_POINT ( 'NONE',  ( -0.3998447049182095037, 0.4754871227241110332, 0.2574803149606298969 ) ) ;
#15326=CARTESIAN_POINT ( 'NONE',  ( -0.4337933494688747671, -0.2502226818840338485, 0.2574827755769819038 ) ) ;
#15327=DIRECTION ( 'NONE',  ( 0.000000000000000000, 1.000000000000000000, 0.000000000000000000 ) ) ;
#15330=B_SPLINE_CURVE_WITH_KNOTS ( 'NONE', 3,
 ( #26727, #7383, #15133, #10304, #17095, #23609 ),
 .UNSPECIFIED., .F., .F.,
 ( 4, 2, 4 ),
 ( 0.000000000000000000, 0.2500000000000000000, 0.5000000000000000000 ),
 .UNSPECIFIED. ) ;
#15349=CARTESIAN_POINT ( 'NONE',  ( 0.000000000000000000, 0.000000000000000000, 0.1771653543307086520 ) ) ;
#15351=CIRCLE ( 'NONE', #20726, 0.7165354330708662012 ) ;
#15378=EDGE_LOOP ( 'NONE', ( #3921, #13867 ) ) ;
#15394=CIRCLE ( 'NONE', #24365, 0.7283464566929134243 ) ;
#15405=B_SPLINE_CURVE_WITH_KNOTS ( 'NONE', 3,
 ( #354, #24051, #23340, #474, #95, #8660 ),
 .UNSPECIFIED., .F., .F.,
 ( 4, 2, 4 ),
 ( 0.3000437156586439613, 0.3015484798814569989, 0.3030532441042709801 ),
 .UNSPECIFIED. ) ;
#15407=CARTESIAN_POINT ( 'NONE',  ( 0.000000000000000000, 0.000000000000000000, 0.1771653543307086520 ) ) ;
#15411=EDGE_LOOP ( 'NONE', ( #18247, #640, #25105, #19674 ) ) ;
#15418=CARTESIAN_POINT ( 'NONE',  ( 0.000000000000000000, 0.000000000000000000, -3.278217716535432842E-17 ) ) ;
#15419=CARTESIAN_POINT ( 'NONE',  ( 0.000000000000000000, 0.6212598425196850238, 0.3059055118110236560 ) ) ;
#15438=DIRECTION ( 'NONE',  ( 0.000000000000000000, 0.000000000000000000, -1.000000000000000000 ) ) ;
#15441=EDGE_CURVE ( 'NONE', #19404, #12816, #16938, .T. ) ;
#15449=DIRECTION ( 'NONE',  ( 0.000000000000000000, 1.000000000000000000, 0.000000000000000000 ) ) ;
#15464=FACE_OUTER_BOUND ( 'NONE', #7181, .T. ) ;
#15471=EDGE_CURVE ( 'NONE', #20711, #798, #13204, .T. ) ;
#15480=ORIENTED_EDGE ( 'NONE', *, *, #13968, .F. ) ;
#15481=CIRCLE ( 'NONE', #12762, 0.7283464566929134243 ) ;
#15484=CARTESIAN_POINT ( 'NONE',  ( 0.0005939837304750000086, 0.5007870493127504208, 0.09685039370078740717 ) ) ;
#15506=CARTESIAN_POINT ( 'NONE',  ( -0.6339803004471820103, 0.1124719464481696296, 0.2359405056191490324 ) ) ;
#15524=EDGE_CURVE ( 'NONE', #4649, #27798, #3833, .T. ) ;
#15531=CARTESIAN_POINT ( 'NONE',  ( -0.2118615749922956593, -0.5840192333899354438, 0.09685039370078740717 ) ) ;
#15532=DIRECTION ( 'NONE',  ( 0.000000000000000000, 1.000000000000000000, 0.000000000000000000 ) ) ;
#15551=VERTEX_POINT ( 'NONE', #8272 ) ;
#15563=CARTESIAN_POINT ( 'NONE',  ( 0.000000000000000000, 0.000000000000000000, 0.3425196850393700809 ) ) ;
#15609=DIRECTION ( 'NONE',  ( 0.000000000000000000, -1.000000000000000000, 0.000000000000000000 ) ) ;
#15610=DIRECTION ( 'NONE',  ( 0.000000000000000000, 1.000000000000000000, 0.000000000000000000 ) ) ;
#15611=ADVANCED_FACE ( 'NONE', ( #14098 ), #25495, .F. ) ;
#15613=VERTEX_POINT ( 'NONE', #10129 ) ;
#15623=CARTESIAN_POINT ( 'NONE',  ( 0.000000000000000000, 0.000000000000000000, 0.2574803149606298969 ) ) ;
#15636=EDGE_CURVE ( 'NONE', #6679, #21791, #12410, .T. ) ;
#15639=VECTOR ( 'NONE', #2094, 39.37007874015748143 ) ;
#15648=EDGE_CURVE ( 'NONE', #13218, #2702, #18957, .T. ) ;
#15670=( NAMED_UNIT ( * ) SI_UNIT ( $, .STERADIAN. ) SOLID_ANGLE_UNIT ( ) ) ;
#15673=EDGE_LOOP ( 'NONE', ( #17975, #14319, #23958, #26617 ) ) ;
#15674=CARTESIAN_POINT ( 'NONE',  ( -4.821444091131312140E-17, -0.3937007874015748254, 0.3425196850393700809 ) ) ;
#15683=DIRECTION ( 'NONE',  ( 0.000000000000000000, -1.000000000000000000, 0.000000000000000000 ) ) ;
#15715=CARTESIAN_POINT ( 'NONE',  ( 0.6119360453657027854, 0.1072290460172409393, 0.2574803149606298969 ) ) ;
#15725=CARTESIAN_POINT ( 'NONE',  ( -0.4930758245789425009, 0.08754571829529331217, 0.2574803149606298969 ) ) ;
#15735=CARTESIAN_POINT ( 'NONE',  ( 0.4078284417489183022, 0.4849914877866832175, 0.2481708550941282843 ) ) ;
#15736=CARTESIAN_POINT ( 'NONE',  ( -0.0006681923949012172652, 0.6336721034116280515, 0.2481708550951330083 ) ) ;
#15761=AXIS2_PLACEMENT_3D ( 'NONE', #4145, #19253, #12478 ) ;
#15777=ORIENTED_EDGE ( 'NONE', *, *, #15822, .F. ) ;
#15792=CARTESIAN_POINT ( 'NONE',  ( -0.5378064472800889728, -0.3110113600220764107, 0.2574819594177527593 ) ) ;
#15797=VERTEX_POINT ( 'NONE', #146 ) ;
#15798=ORIENTED_EDGE ( 'NONE', *, *, #17839, .T. ) ;
#15816=CARTESIAN_POINT ( 'NONE',  ( -2.183966630091013010E-17, 0.6212598425196852459, 0.09684793308443542803 ) ) ;
#15818=DIRECTION ( 'NONE',  ( 0.000000000000000000, 0.000000000000000000, 1.000000000000000000 ) ) ;
#15822=EDGE_CURVE ( 'NONE', #24679, #27463, #7433, .T. ) ;
#15826=CARTESIAN_POINT ( 'NONE',  ( 0.4126915023386704684, -0.2375990494935494579, 0.1212655228829027515 ) ) ;
#15834=ORIENTED_EDGE ( 'NONE', *, *, #25396, .F. ) ;
#15838=CARTESIAN_POINT ( 'NONE',  ( 0.4339912984563291110, -0.2498791196563492356, 0.2574803149606298969 ) ) ;
#15859=CARTESIAN_POINT ( 'NONE',  ( 0.4233199042360576425, 0.5034331896086758906, 0.1461456498285838845 ) ) ;
#15863=DIRECTION ( 'NONE',  ( 0.1736481776669299981, -0.9848077530122081313, 0.000000000000000000 ) ) ;
#15865=ORIENTED_EDGE ( 'NONE', *, *, #18612, .F. ) ;
#15868=VERTEX_POINT ( 'NONE', #22927 ) ;
#15878=EDGE_CURVE ( 'NONE', #3924, #8098, #10618, .T. ) ;
#15881=CIRCLE ( 'NONE', #21301, 0.3937007874015748254 ) ;
#15885=CARTESIAN_POINT ( 'NONE',  ( 0.0003954787107570253350, 0.5007872847596378518, 0.09684874903502814492 ) ) ;
#15886=ORIENTED_EDGE ( 'NONE', *, *, #5062, .F. ) ;
#15889=CARTESIAN_POINT ( 'NONE',  ( -2.184900367198595585E-17, 0.6212598425196850238, 0.2574827755769818483 ) ) ;
#15905=VERTEX_POINT ( 'NONE', #2985 ) ;
#15911=ORIENTED_EDGE ( 'NONE', *, *, #12607, .T. ) ;
#15930=DIRECTION ( 'NONE',  ( 0.000000000000000000, 1.000000000000000000, 0.000000000000000000 ) ) ;
#15940=EDGE_CURVE ( 'NONE', #8070, #24688, #1823, .T. ) ;
#15946=ORIENTED_EDGE ( 'NONE', *, *, #21977, .F. ) ;
#15965=ORIENTED_EDGE ( 'NONE', *, *, #22642, .T. ) ;
#15966=DIRECTION ( 'NONE',  ( 0.000000000000000000, 0.000000000000000000, 1.000000000000000000 ) ) ;
#16006=CARTESIAN_POINT ( 'NONE',  ( -0.4333973147258542991, -0.2509079296564011852, 0.09685039370078740717 ) ) ;
#16013=SPHERICAL_SURFACE ( 'NONE', #13818, 0.1003956692913385851 ) ;
#16020=CARTESIAN_POINT ( 'NONE',  ( -0.4932821129636645874, 0.08637579872942342807, 0.09685039370078740717 ) ) ;
#16029=B_SPLINE_CURVE_WITH_KNOTS ( 'NONE', 3,
 ( #1240, #1369, #13950, #7875, #7737, #20303 ),
 .UNSPECIFIED., .F., .F.,
 ( 4, 2, 4 ),
 ( 0.5000000000000000000, 0.7500000000000000000, 1.000000000000000000 ),
 .UNSPECIFIED. ) ;
#16033=AXIS2_PLACEMENT_3D ( 'NONE', #17551, #19251, #15449 ) ;
#16073=CARTESIAN_POINT ( 'NONE',  ( -0.5376957092749378164, -0.3112026930392873814, 0.2574803149606298969 ) ) ;
#16082=VERTEX_POINT ( 'NONE', #14770 ) ;
#16083=CARTESIAN_POINT ( 'NONE',  ( -0.3223547283257516272, 0.3832433309296771617, 0.09685039370078740717 ) ) ;
#16091=EDGE_LOOP ( 'NONE', ( #5347, #20962, #25119, #17034, #26054 ) ) ;
#16117=CARTESIAN_POINT ( 'NONE',  ( -0.2208527687073504053, -0.6048181665964218467, 0.2359405056213304541 ) ) ;
#16123=ORIENTED_EDGE ( 'NONE', *, *, #17628, .F. ) ;
#16131=CARTESIAN_POINT ( 'NONE',  ( 0.4337933494688747671, -0.2502226818840338485, 0.2574827755769819038 ) ) ;
#16144=ADVANCED_FACE ( 'NONE', ( #4681 ), #6406, .F. ) ;
#16151=FACE_OUTER_BOUND ( 'NONE', #21824, .T. ) ;
#16164=ORIENTED_EDGE ( 'NONE', *, *, #21663, .T. ) ;
#16168=CIRCLE ( 'NONE', #16624, 0.5007874015748031704 ) ;
#16169=CARTESIAN_POINT ( 'NONE',  ( 0.3986320731132086959, -0.2308081338369904478, 0.1771653543307089018 ) ) ;
#16178=ORIENTED_EDGE ( 'NONE', *, *, #19204, .F. ) ;
#16181=AXIS2_PLACEMENT_3D ( 'NONE', #4821, #13437, #23657 ) ;
#16191=ORIENTED_EDGE ( 'NONE', *, *, #5518, .T. ) ;
#16200=ORIENTED_EDGE ( 'NONE', *, *, #13134, .T. ) ;
#16201=ORIENTED_EDGE ( 'NONE', *, *, #11636, .F. ) ;
#16210=ADVANCED_FACE ( 'NONE', ( #13029 ), #17387, .F. ) ;
#16213=CARTESIAN_POINT ( 'NONE',  ( 0.000000000000000000, 0.000000000000000000, 0.1771653543307086520 ) ) ;
#16214=CARTESIAN_POINT ( 'NONE',  ( -0.4930758245789425009, 0.08754571829529331217, 0.09685039370078740717 ) ) ;
#16216=CARTESIAN_POINT ( 'NONE',  ( 0.3220512119205940493, 0.3834984712787528061, 0.09684793308443542803 ) ) ;
#16218=CARTESIAN_POINT ( 'NONE',  ( -0.4858607088160732390, -0.2805118110236220486, 0.1771653543307086520 ) ) ;
#16229=FACE_OUTER_BOUND ( 'NONE', #17870, .T. ) ;
#16236=CARTESIAN_POINT ( 'NONE',  ( 0.4333973147258542991, -0.2509079296564015737, 0.09685039370078740717 ) ) ;
#16259=ORIENTED_EDGE ( 'NONE', *, *, #14708, .F. ) ;
#16269=EDGE_CURVE ( 'NONE', #15613, #9254, #24354, .T. ) ;
#16284=CARTESIAN_POINT ( 'NONE',  ( 0.000000000000000000, 0.000000000000000000, 0.3425196850393700809 ) ) ;
#16298=ORIENTED_EDGE ( 'NONE', *, *, #16918, .F. ) ;
#16299=CARTESIAN_POINT ( 'NONE',  ( 0.3606190329934327310, 0.4297690281277732338, 0.2775610236220472093 ) ) ;
#16300=ORIENTED_EDGE ( 'NONE', *, *, #26119, .F. ) ;
#16303=CARTESIAN_POINT ( 'NONE',  ( 0.5491102354219981052, -0.3162573801175324051, 0.1061598535667657994 ) ) ;
#16318=EDGE_CURVE ( 'NONE', #5816, #6596, #14919, .T. ) ;
#16326=EDGE_LOOP ( 'NONE', ( #21034, #23314, #20911, #25019, #1167, #16333 ) ) ;
#16330=PRODUCT_DEFINITION_SHAPE ( 'NONE', 'NONE',  #10324 ) ;
#16332=VERTEX_POINT ( 'NONE', #22194 ) ;
#16333=ORIENTED_EDGE ( 'NONE', *, *, #4377, .F. ) ;
#16353=VERTEX_POINT ( 'NONE', #5388 ) ;
#16354=CARTESIAN_POINT ( 'NONE',  ( -0.5382469622847110280, -0.3102483656525752420, 0.2574819594177527593 ) ) ;
#16357=CARTESIAN_POINT ( 'NONE',  ( 6.147461752294700483E-18, 0.5610236220472440971, 0.07676968503937006694 ) ) ;
#16358=DIRECTION ( 'NONE',  ( 0.000000000000000000, -1.000000000000000000, 0.000000000000000000 ) ) ;
#16366=CARTESIAN_POINT ( 'NONE',  ( 0.2118615749922956593, -0.5840192333899354438, 0.09685039370078740717 ) ) ;
#16373=ADVANCED_FACE ( 'NONE', ( #7092 ), #13572, .T. ) ;
#16375=ORIENTED_EDGE ( 'NONE', *, *, #17268, .T. ) ;
#16398=CIRCLE ( 'NONE', #4233, 0.5007874015748031704 ) ;
#16406=CARTESIAN_POINT ( 'NONE',  ( -0.1709077104829875848, -0.4707213777573787672, 0.2574819596263889787 ) ) ;
#16420=CARTESIAN_POINT ( 'NONE',  ( 0.000000000000000000, 0.000000000000000000, 0.1771653543307086520 ) ) ;
#16441=EDGE_LOOP ( 'NONE', ( #25538, #18517, #980, #13375 ) ) ;
#16448=CIRCLE ( 'NONE', #24111, 0.5007874015748031704 ) ;
#16451=AXIS2_PLACEMENT_3D ( 'NONE', #6092, #12841, #20908 ) ;
#16455=VERTEX_POINT ( 'NONE', #20640 ) ;
#16474=DIRECTION ( 'NONE',  ( 0.000000000000000000, 1.000000000000000000, 0.000000000000000000 ) ) ;
#16485=CARTESIAN_POINT ( 'NONE',  ( -0.0005696707463070112927, 0.4606295689977898400, 0.1771653543307085965 ) ) ;
#16510=DIRECTION ( 'NONE',  ( 1.000000000000000000, 0.000000000000000000, 0.000000000000000000 ) ) ;
#16532=AXIS2_PLACEMENT_3D ( 'NONE', #693, #13536, #8888 ) ;
#16556=( GEOMETRIC_REPRESENTATION_CONTEXT ( 3 ) GLOBAL_UNCERTAINTY_ASSIGNED_CONTEXT ( ( #25134 ) ) GLOBAL_UNIT_ASSIGNED_CONTEXT ( ( #14651, #7992, #10226 ) ) REPRESENTATION_CONTEXT ( 'NONE', 'WORKASPACE' ) ) ;
#16558=ORIENTED_EDGE ( 'NONE', *, *, #23544, .F. ) ;
#16598=DIRECTION ( 'NONE',  ( 0.000000000000000000, 0.000000000000000000, 1.000000000000000000 ) ) ;
#16615=TOROIDAL_SURFACE ( 'NONE', #26983, 0.5610236220472440971, 0.1003937007874015908 ) ;
#16624=AXIS2_PLACEMENT_3D ( 'NONE', #2688, #18208, #11875 ) ;
#16625=FACE_OUTER_BOUND ( 'NONE', #15673, .T. ) ;
#16626=ADVANCED_FACE ( 'NONE', ( #8623, #10880 ), #17105, .T. ) ;
#16631=PLANE ( 'NONE',  #10316 ) ;
#16633=SPHERICAL_SURFACE ( 'NONE', #17798, 0.1003956692913385851 ) ;
#16635=DIRECTION ( 'NONE',  ( 1.000000000000000000, 0.000000000000000000, 0.000000000000000000 ) ) ;
#16636=CARTESIAN_POINT ( 'NONE',  ( -0.2173565190932491564, -0.5952284643155388855, 0.1061598535666244958 ) ) ;
#16644=EDGE_LOOP ( 'NONE', ( #1698, #18489, #2248, #3929, #21178, #23298, #5787, #14182 ) ) ;
#16646=CARTESIAN_POINT ( 'NONE',  ( 0.4790450267257945760, 0.08506312950213980317, 0.2467937633157138710 ) ) ;
#16656=ORIENTED_EDGE ( 'NONE', *, *, #8429, .T. ) ;
#16660=CARTESIAN_POINT ( 'NONE',  ( 0.2118615749922956593, -0.5840192333899354438, 0.09685039370078740717 ) ) ;
#16661=FACE_OUTER_BOUND ( 'NONE', #12163, .T. ) ;
#16675=CARTESIAN_POINT ( 'NONE',  ( -0.4858607088160732390, -0.2805118110236220486, 0.1771653543307086520 ) ) ;
#16677=B_SPLINE_CURVE_WITH_KNOTS ( 'NONE', 3,
 ( #8601, #6769, #7037, #19893, #168, #15531 ),
 .UNSPECIFIED., .F., .F.,
 ( 4, 2, 4 ),
 ( 0.3108507187342960387, 0.3125269569790680158, 0.3142031952238389936 ),
 .UNSPECIFIED. ) ;
#16678=ORIENTED_EDGE ( 'NONE', *, *, #4830, .F. ) ;
#16680=DIRECTION ( 'NONE',  ( 0.000000000000000000, 0.000000000000000000, -1.000000000000000000 ) ) ;
#16683=CARTESIAN_POINT ( 'NONE',  ( -0.3215969074633125979, 0.3838795254899315390, 0.09684874903502814492 ) ) ;
#16685=B_SPLINE_CURVE_WITH_KNOTS ( 'NONE', 3,
 ( #6382, #8500, #23629, #4265, #24664, #5176, #11680, #24394, #3189, #22563 ),
 .UNSPECIFIED., .F., .F.,
 ( 4, 2, 2, 2, 4 ),
 ( 0.000000000000000000, 0.2499999999999997224, 0.4999999999999994449, 0.7499999999999996669, 1.000000000000000000 ),
 .UNSPECIFIED. ) ;
#16688=ORIENTED_EDGE ( 'NONE', *, *, #13139, .T. ) ;
#16691=CARTESIAN_POINT ( 'NONE',  ( -7.608238775805210269E-17, -0.6212598425196850238, 0.2574803149606298969 ) ) ;
#16697=CARTESIAN_POINT ( 'NONE',  ( -0.1707210962531915677, -0.4707890492249701131, 0.09685039370078740717 ) ) ;
#16722=DIRECTION ( 'NONE',  ( 1.224646799147353207E-16, 1.000000000000000000, -0.000000000000000000 ) ) ;
#16723=ORIENTED_EDGE ( 'NONE', *, *, #10194, .T. ) ;
#16725=ORIENTED_EDGE ( 'NONE', *, *, #21514, .T. ) ;
#16739=LENGTH_MEASURE_WITH_UNIT ( LENGTH_MEASURE( 0.02539999999999999897 ), #27202 ) ;
#16751=CARTESIAN_POINT ( 'NONE',  ( -0.1918813796216842782, -0.5271897577243779276, 0.2775610236220472093 ) ) ;
#16765=CARTESIAN_POINT ( 'NONE',  ( -0.7283464566929135353, 8.919671568592928630E-17, 0.01181102362204724393 ) ) ;
#16770=CARTESIAN_POINT ( 'NONE',  ( -0.0005710523241063101023, 0.4632828964882294565, 0.1494804572083954508 ) ) ;
#16773=EDGE_CURVE ( 'NONE', #22917, #12919, #22089, .T. ) ;
#16784=CARTESIAN_POINT ( 'NONE',  ( -0.4078284417495566250, 0.4849914877874417218, 0.2481708550933849622 ) ) ;
#16786=B_SPLINE_CURVE_WITH_KNOTS ( 'NONE', 3,
 ( #7760, #11844, #14112, #20466, #7617, #16236 ),
 .UNSPECIFIED., .F., .F.,
 ( 4, 2, 4 ),
 ( 0.3000437156586439613, 0.3015484798814569989, 0.3030532441042709801 ),
 .UNSPECIFIED. ) ;
#16793=CARTESIAN_POINT ( 'NONE',  ( -0.5383572925355968319, -0.3100567972183898013, 0.09685039370078740717 ) ) ;
#16796=B_SPLINE_CURVE_WITH_KNOTS ( 'NONE', 3,
 ( #659, #15108, #10987, #23720, #8857, #4354 ),
 .UNSPECIFIED., .F., .F.,
 ( 4, 2, 4 ),
 ( 0.3108507187342950395, 0.3125269569790670166, 0.3142031952238389936 ),
 .UNSPECIFIED. ) ;
#16805=TOROIDAL_SURFACE ( 'NONE', #4602, 0.5610236220472440971, 0.1003937007874015908 ) ;
#16854=TOROIDAL_SURFACE ( 'NONE', #8740, 0.7165354330708662012, 0.01181102362204724393 ) ;
#16856=ADVANCED_FACE ( 'NONE', ( #18855, #27502 ), #23268, .T. ) ;
#16872=CYLINDRICAL_SURFACE ( 'NONE', #1816, 0.6212598425196850238 ) ;
#16880=ORIENTED_EDGE ( 'NONE', *, *, #15441, .F. ) ;
#16888=DIRECTION ( 'NONE',  ( -0.9396926207859082059, -0.3420201433256690460, 0.000000000000000000 ) ) ;
#16890=CARTESIAN_POINT ( 'NONE',  ( -0.3056525133683296036, 0.3651631491442455246, 0.1212655228852408396 ) ) ;
#16892=AXIS2_PLACEMENT_3D ( 'NONE', #26017, #10903, #2681 ) ;
#16908=CARTESIAN_POINT ( 'NONE',  ( 0.0005939837304750000086, 0.5007870493127504208, 0.2574803149606298969 ) ) ;
#16918=EDGE_CURVE ( 'NONE', #730, #27022, #14910, .T. ) ;
#16921=CARTESIAN_POINT ( 'NONE',  ( 0.000000000000000000, 0.000000000000000000, 0.09685039370078740717 ) ) ;
#16938=CIRCLE ( 'NONE', #11055, 0.4606299212598425341 ) ;
#16946=DIRECTION ( 'NONE',  ( 0.000000000000000000, -1.000000000000000000, 0.000000000000000000 ) ) ;
#16973=CARTESIAN_POINT ( 'NONE',  ( -0.4792483803617587634, 0.08390985360245291347, 0.2467937632999436248 ) ) ;
#16979=VERTEX_POINT ( 'NONE', #16169 ) ;
#16983=DIRECTION ( 'NONE',  ( 0.000000000000000000, 0.000000000000000000, 1.000000000000000000 ) ) ;
#16992=ADVANCED_FACE ( 'NONE', ( #22656 ), #4057, .F. ) ;
#16996=CARTESIAN_POINT ( 'NONE',  ( -0.3986320731132244610, -0.2308081338369635804, 0.1771653543307087630 ) ) ;
#17000=B_SPLINE_CURVE_WITH_KNOTS ( 'NONE', 3,
 ( #27580, #8222, #19658, #327, #4537, #21636, #13142, #13007, #19785, #19228 ),
 .UNSPECIFIED., .F., .F.,
 ( 4, 2, 2, 2, 4 ),
 ( 0.000000000000000000, 0.2500000000000000000, 0.5000000000000000000, 0.7500000000000000000, 1.000000000000000000 ),
 .UNSPECIFIED. ) ;
#17004=CARTESIAN_POINT ( 'NONE',  ( 0.1718374205099799101, -0.4703827404237102550, 0.09685039370078740717 ) ) ;
#17025=CARTESIAN_POINT ( 'NONE',  ( 0.000000000000000000, 0.000000000000000000, 0.09685039370078740717 ) ) ;
#17026=CARTESIAN_POINT ( 'NONE',  ( -0.2973550541829020344, 0.3552623538055160179, 0.1494804572073591964 ) ) ;
#17034=ORIENTED_EDGE ( 'NONE', *, *, #13968, .T. ) ;
#17044=DIRECTION ( 'NONE',  ( 0.000000000000000000, 0.000000000000000000, -1.000000000000000000 ) ) ;
#17048=ADVANCED_FACE ( 'NONE', ( #22945 ), #2683, .F. ) ;
#17053=CARTESIAN_POINT ( 'NONE',  ( -0.0005789383928811193264, 0.4762008496958949344, 0.1212655228861402035 ) ) ;
#17060=ORIENTED_EDGE ( 'NONE', *, *, #17844, .T. ) ;
#17064=CARTESIAN_POINT ( 'NONE',  ( 0.4561454261165569513, 0.08101060747777377724, 0.2048502514975752697 ) ) ;
#17066=CIRCLE ( 'NONE', #2176, 0.6212598425196850238 ) ;
#17070=VERTEX_POINT ( 'NONE', #17004 ) ;
#17081=CARTESIAN_POINT ( 'NONE',  ( 0.7165354330708662012, 0.000000000000000000, 0.01181102362204724393 ) ) ;
#17089=CIRCLE ( 'NONE', #12571, 0.1003956692913385851 ) ;
#17095=CARTESIAN_POINT ( 'NONE',  ( 0.1580799066051611357, -0.4326553680327475671, 0.1903859678396761790 ) ) ;
#17105=PLANE ( 'NONE',  #24342 ) ;
#17113=DIRECTION ( 'NONE',  ( 0.000000000000000000, 1.000000000000000000, 0.000000000000000000 ) ) ;
#17116=CARTESIAN_POINT ( 'NONE',  ( -0.1710938124795999826, -0.4706537664821763833, 0.09684793308443542803 ) ) ;
#17129=ADVANCED_FACE ( 'NONE', ( #18970 ), #16872, .F. ) ;
#17139=DIRECTION ( 'NONE',  ( 1.000000000000000000, 0.000000000000000000, 0.000000000000000000 ) ) ;
#17140=CARTESIAN_POINT ( 'NONE',  ( 0.3988311005573134116, 0.4763376377694984454, 0.09685039370078740717 ) ) ;
#17148=VERTEX_POINT ( 'NONE', #5996 ) ;
#17165=CARTESIAN_POINT ( 'NONE',  ( 0.4055118110236220486, 0.000000000000000000, 0.01181102362204724393 ) ) ;
#17174=CARTESIAN_POINT ( 'NONE',  ( -0.5484420430269733027, -0.3174147232946766817, 0.1061598535666647691 ) ) ;
#17179=CARTESIAN_POINT ( 'NONE',  ( 0.5525004126151165096, 0.09742072959660433296, 0.1771653543307086520 ) ) ;
#17184=DIRECTION ( 'NONE',  ( 0.000000000000000000, 0.000000000000000000, 1.000000000000000000 ) ) ;
#17189=ORIENTED_EDGE ( 'NONE', *, *, #23042, .T. ) ;
#17192=CARTESIAN_POINT ( 'NONE',  ( 0.4932821129636645874, 0.08637579872942321990, 0.09685039370078740717 ) ) ;
#17201=B_SPLINE_CURVE_WITH_KNOTS ( 'NONE', 3,
 ( #27190, #12484, #5718, #10077, #23385, #25056 ),
 .UNSPECIFIED., .F., .F.,
 ( 4, 2, 4 ),
 ( 0.9359046326923009529, 0.9375808709372039917, 0.9392571091821080298 ),
 .UNSPECIFIED. ) ;
#17207=EDGE_CURVE ( 'NONE', #22691, #14646, #17593, .T. ) ;
#17212=ORIENTED_EDGE ( 'NONE', *, *, #2233, .T. ) ;
#17238=FACE_OUTER_BOUND ( 'NONE', #19909, .T. ) ;
#17244=CARTESIAN_POINT ( 'NONE',  ( -0.4339912984563299436, -0.2498791196563492356, 0.09685039370078740717 ) ) ;
#17267=AXIS2_PLACEMENT_3D ( 'NONE', #14881, #8489, #17113 ) ;
#17268=EDGE_CURVE ( 'NONE', #26549, #23101, #19335, .T. ) ;
#17285=VERTEX_POINT ( 'NONE', #9062 ) ;
#17289=EDGE_CURVE ( 'NONE', #26710, #11052, #1468, .T. ) ;
#17319=TOROIDAL_SURFACE ( 'NONE', #5117, 0.7165354330708662012, 0.01181102362204724393 ) ;
#17321=CARTESIAN_POINT ( 'NONE',  ( -0.6118597084614586512, 0.1076640027107653580, 0.2574827755769819038 ) ) ;
#17340=ORIENTED_EDGE ( 'NONE', *, *, #10914, .T. ) ;
#17342=SPHERICAL_SURFACE ( 'NONE', #14087, 0.1003956692913385851 ) ;
#17345=VERTEX_POINT ( 'NONE', #21793 ) ;
#17351=ORIENTED_EDGE ( 'NONE', *, *, #14410, .T. ) ;
#17376=CARTESIAN_POINT ( 'NONE',  ( 0.000000000000000000, 0.000000000000000000, 0.09685039370078740717 ) ) ;
#17383=DIRECTION ( 'NONE',  ( 1.000000000000000000, 0.000000000000000000, 0.000000000000000000 ) ) ;
#17387=TOROIDAL_SURFACE ( 'NONE', #5189, 0.5610236220472440971, 0.1003937007874015908 ) ;
#17393=ADVANCED_FACE ( 'NONE', ( #20502 ), #5291, .F. ) ;
#17400=AXIS2_PLACEMENT_3D ( 'NONE', #12176, #6776, #4101 ) ;
#17413=CARTESIAN_POINT ( 'NONE',  ( -0.4335958738490826581, -0.2505647196907692664, 0.2574827755769819038 ) ) ;
#17414=DIRECTION ( 'NONE',  ( 0.000000000000000000, 1.000000000000000000, 0.000000000000000000 ) ) ;
#17416=ORIENTED_EDGE ( 'NONE', *, *, #27539, .F. ) ;
#17443=CARTESIAN_POINT ( 'NONE',  ( 0.000000000000000000, 0.000000000000000000, 0.1771653543307086520 ) ) ;
#17444=ORIENTED_EDGE ( 'NONE', *, *, #21977, .T. ) ;
#17447=EDGE_CURVE ( 'NONE', #18606, #26549, #10513, .T. ) ;
#17460=EDGE_CURVE ( 'NONE', #21648, #19560, #22327, .T. ) ;
#17465=CARTESIAN_POINT ( 'NONE',  ( 0.4792483803810960730, 0.08390985360584736485, 0.1075369453467489578 ) ) ;
#17474=CARTESIAN_POINT ( 'NONE',  ( -8.919671568592927398E-17, -0.7283464566929134243, 0.01181102362204724393 ) ) ;
#17485=CARTESIAN_POINT ( 'NONE',  ( 0.4333973147258542991, -0.2509079296564015737, 0.09685039370078740717 ) ) ;
#17492=ADVANCED_FACE ( 'NONE', ( #10171 ), #2581, .F. ) ;
#17505=ORIENTED_EDGE ( 'NONE', *, *, #17289, .T. ) ;
#17509=CARTESIAN_POINT ( 'NONE',  ( -0.1634143070176771462, -0.4472844159263525965, 0.1212655228098387938 ) ) ;
#17523=CARTESIAN_POINT ( 'NONE',  ( 0.000000000000000000, 0.000000000000000000, 0.3543307086614173040 ) ) ;
#17539=B_SPLINE_CURVE_WITH_KNOTS ( 'NONE', 3,
 ( #9764, #27430, #3386, #8083, #14599, #16697 ),
 .UNSPECIFIED., .F., .F.,
 ( 4, 2, 4 ),
 ( 0.5000000000000000000, 0.7500000000000000000, 1.000000000000000000 ),
 .UNSPECIFIED. ) ;
#17551=CARTESIAN_POINT ( 'NONE',  ( 0.000000000000000000, 0.000000000000000000, 0.1771653543307086520 ) ) ;
#17573=CARTESIAN_POINT ( 'NONE',  ( -0.0006812437162517212324, 0.6577569867587390595, 0.2081850588307845862 ) ) ;
#17584=DIRECTION ( 'NONE',  ( -0.9396926207859083169, 0.3420201433256692125, 0.000000000000000000 ) ) ;
#17589=DIRECTION ( 'NONE',  ( 0.000000000000000000, 0.000000000000000000, 1.000000000000000000 ) ) ;
#17593=CIRCLE ( 'NONE', #4083, 0.3937007874015748254 ) ;
#17594=CIRCLE ( 'NONE', #4965, 0.6212598425196850238 ) ;
#17595=ORIENTED_EDGE ( 'NONE', *, *, #13073, .F. ) ;
#17597=DIRECTION ( 'NONE',  ( 0.7660444431189777914, -0.6427876096865396960, 0.000000000000000000 ) ) ;
#17620=CARTESIAN_POINT ( 'NONE',  ( -0.1918813796216842782, -0.5271897577243779276, 0.1771653543307086520 ) ) ;
#17628=EDGE_CURVE ( 'NONE', #14152, #20711, #23985, .T. ) ;
#17643=B_SPLINE_CURVE_WITH_KNOTS ( 'NONE', 3,
 ( #621, #2986, #9343, #2847, #11485, #17954, #22363, #26588, #9488, #18085 ),
 .UNSPECIFIED., .F., .F.,
 ( 4, 2, 2, 2, 4 ),
 ( 0.000000000000000000, 0.2500000000000000000, 0.5000000000000000000, 0.7500000000000000000, 1.000000000000000000 ),
 .UNSPECIFIED. ) ;
#17647=CARTESIAN_POINT ( 'NONE',  ( 0.000000000000000000, 0.5610236220472440971, 0.3543307086614173040 ) ) ;
#17648=EDGE_CURVE ( 'NONE', #4007, #15131, #1271, .T. ) ;
#17698=CARTESIAN_POINT ( 'NONE',  ( -0.1658556822967069411, -0.4573967274743634404, 0.2467937633334012226 ) ) ;
#17711=EDGE_CURVE ( 'NONE', #15797, #290, #7463, .T. ) ;
#17717=CARTESIAN_POINT ( 'NONE',  ( 0.6476458834291769495, 0.1148891961919920740, 0.1461456498338012666 ) ) ;
#17722=AXIS2_PLACEMENT_3D ( 'NONE', #11191, #473, #15327 ) ;
#17723=VERTEX_POINT ( 'NONE', #13547 ) ;
#17731=AXIS2_PLACEMENT_3D ( 'NONE', #1272, #15966, #9587 ) ;
#17755=EDGE_CURVE ( 'NONE', #17779, #27463, #1408, .T. ) ;
#17769=EDGE_LOOP ( 'NONE', ( #22791, #25944, #5021, #15777 ) ) ;
#17771=ORIENTED_EDGE ( 'NONE', *, *, #9457, .T. ) ;
#17772=AXIS2_PLACEMENT_3D ( 'NONE', #22636, #7810, #7378 ) ;
#17775=EDGE_LOOP ( 'NONE', ( #15965, #20350, #10608, #26165, #3732, #21865 ) ) ;
#17779=VERTEX_POINT ( 'NONE', #2797 ) ;
#17793=CARTESIAN_POINT ( 'NONE',  ( 0.3992017438595160117, -0.2298214351608009742, 0.1639447408809755480 ) ) ;
#17798=AXIS2_PLACEMENT_3D ( 'NONE', #25248, #11687, #20308 ) ;
#17801=DIRECTION ( 'NONE',  ( 0.000000000000000000, 0.000000000000000000, 1.000000000000000000 ) ) ;
#17807=EDGE_CURVE ( 'NONE', #6679, #10869, #3093, .T. ) ;
#17812=EDGE_CURVE ( 'NONE', #21446, #9472, #17066, .T. ) ;
#17814=FACE_OUTER_BOUND ( 'NONE', #14904, .T. ) ;
#17818=EDGE_CURVE ( 'NONE', #18356, #2702, #5797, .T. ) ;
#17822=CARTESIAN_POINT ( 'NONE',  ( 0.6117448998508603353, 0.1083144418130616154, 0.2574819594177531479 ) ) ;
#17826=ORIENTED_EDGE ( 'NONE', *, *, #19694, .T. ) ;
#17831=CARTESIAN_POINT ( 'NONE',  ( 0.4143937130589223639, 0.4928070724598411778, 0.1183902030385255016 ) ) ;
#17832=CIRCLE ( 'NONE', #2951, 0.01181102362204724393 ) ;
#17838=ORIENTED_EDGE ( 'NONE', *, *, #17460, .T. ) ;
#17839=EDGE_CURVE ( 'NONE', #7282, #11900, #20663, .T. ) ;
#17844=EDGE_CURVE ( 'NONE', #24177, #25476, #27395, .T. ) ;
#17848=CARTESIAN_POINT ( 'NONE',  ( 0.6117062799105531523, 0.1085321106658064944, 0.2574803149606298969 ) ) ;
#17849=EDGE_LOOP ( 'NONE', ( #26633, #18764 ) ) ;
#17850=CARTESIAN_POINT ( 'NONE',  ( 0.4858607088160724063, -0.2805118110236220486, 0.07676968503937006694 ) ) ;
#17870=EDGE_LOOP ( 'NONE', ( #13214, #22530 ) ) ;
#17871=VERTEX_POINT ( 'NONE', #5932 ) ;
#17881=AXIS2_PLACEMENT_3D ( 'NONE', #22825, #9955, #5737 ) ;
#17882=CARTESIAN_POINT ( 'NONE',  ( 0.3223547283257516272, 0.3832433309296771617, 0.09685039370078740717 ) ) ;
#17890=( NAMED_UNIT ( * ) PLANE_ANGLE_UNIT ( ) SI_UNIT ( $, .RADIAN. ) ) ;
#17891=VERTEX_POINT ( 'NONE', #25411 ) ;
#17908=CARTESIAN_POINT ( 'NONE',  ( -0.4068047116067418645, 0.4858504993712711162, 0.2481708550942073044 ) ) ;
#17929=VERTEX_POINT ( 'NONE', #17485 ) ;
#17954=CARTESIAN_POINT ( 'NONE',  ( -0.5731455175603529240, -0.3301167833455554423, 0.1616495878887042326 ) ) ;
#17963=CARTESIAN_POINT ( 'NONE',  ( 0.000000000000000000, 0.000000000000000000, 0.3543307086614173040 ) ) ;
#17975=ORIENTED_EDGE ( 'NONE', *, *, #10461, .T. ) ;
#18001=FACE_BOUND ( 'NONE', #24283, .T. ) ;
#18029=ORIENTED_EDGE ( 'NONE', *, *, #1911, .T. ) ;
#18043=ORIENTED_EDGE ( 'NONE', *, *, #19368, .F. ) ;
#18061=EDGE_CURVE ( 'NONE', #6009, #23041, #18404, .T. ) ;
#18080=DIRECTION ( 'NONE',  ( 0.000000000000000000, 0.000000000000000000, 1.000000000000000000 ) ) ;
#18084=CARTESIAN_POINT ( 'NONE',  ( 0.4858607088160724063, -0.2805118110236220486, 0.1771653543307086520 ) ) ;
#18085=CARTESIAN_POINT ( 'NONE',  ( -0.5383572925355968319, -0.3100567972183898013, 0.09685039370078740717 ) ) ;
#18090=ORIENTED_EDGE ( 'NONE', *, *, #7701, .F. ) ;
#18105=DIRECTION ( 'NONE',  ( 0.000000000000000000, -1.000000000000000000, 0.000000000000000000 ) ) ;
#18121=AXIS2_PLACEMENT_3D ( 'NONE', #15349, #24073, #23941 ) ;
#18130=ORIENTED_EDGE ( 'NONE', *, *, #7947, .T. ) ;
#18150=DIRECTION ( 'NONE',  ( 0.000000000000000000, 0.000000000000000000, 1.000000000000000000 ) ) ;
#18156=CARTESIAN_POINT ( 'NONE',  ( -0.5381367953593149123, -0.3104394140547397374, 0.2574827755769819038 ) ) ;
#18160=CIRCLE ( 'NONE', #6489, 0.3937007874015748254 ) ;
#18164=ORIENTED_EDGE ( 'NONE', *, *, #16318, .F. ) ;
#18178=DIRECTION ( 'NONE',  ( 0.000000000000000000, 0.000000000000000000, -1.000000000000000000 ) ) ;
#18179=AXIS2_PLACEMENT_3D ( 'NONE', #16213, #24816, #20588 ) ;
#18181=DIRECTION ( 'NONE',  ( 0.000000000000000000, 1.000000000000000000, 0.000000000000000000 ) ) ;
#18184=CARTESIAN_POINT ( 'NONE',  ( -0.1580799066051628565, -0.4326553680327470675, 0.1903859678385282639 ) ) ;
#18188=DIRECTION ( 'NONE',  ( 1.000000000000000000, 0.000000000000000000, 0.000000000000000000 ) ) ;
#18200=DIRECTION ( 'NONE',  ( 0.1736481776669299426, -0.9848077530122081313, 0.000000000000000000 ) ) ;
#18208=DIRECTION ( 'NONE',  ( 0.000000000000000000, 0.000000000000000000, 1.000000000000000000 ) ) ;
#18236=CARTESIAN_POINT ( 'NONE',  ( 0.1714649452450068834, -0.4705186852026070898, 0.2574827755769819038 ) ) ;
#18247=ORIENTED_EDGE ( 'NONE', *, *, #17807, .T. ) ;
#18255=ORIENTED_EDGE ( 'NONE', *, *, #3464, .T. ) ;
#18256=CIRCLE ( 'NONE', #17400, 0.1003956692913385712 ) ;
#18292=B_SPLINE_CURVE_WITH_KNOTS ( 'NONE', 3,
 ( #16485, #8301, #16770, #17053, #14387, #18873 ),
 .UNSPECIFIED., .F., .F.,
 ( 4, 2, 4 ),
 ( 0.5000000000000000000, 0.7500000000000000000, 1.000000000000000000 ),
 .UNSPECIFIED. ) ;
#18294=FACE_OUTER_BOUND ( 'NONE', #12686, .T. ) ;
#18297=CARTESIAN_POINT ( 'NONE',  ( -0.2131049448084480213, -0.5835666837866708700, 0.2574803149606298969 ) ) ;
#18303=CARTESIAN_POINT ( 'NONE',  ( -0.5381367953593070297, -0.3104394140547547809, 0.09684793308443542803 ) ) ;
#18306=CARTESIAN_POINT ( 'NONE',  ( 0.2982299571078434464, 0.3545282230955180136, 0.2048502514855274625 ) ) ;
#18307=AXIS2_PLACEMENT_3D ( 'NONE', #17376, #1843, #27704 ) ;
#18330=DIRECTION ( 'NONE',  ( 0.000000000000000000, 0.000000000000000000, 1.000000000000000000 ) ) ;
#18333=AXIS2_PLACEMENT_3D ( 'NONE', #22701, #2031, #10643 ) ;
#18345=ADVANCED_FACE ( 'NONE', ( #13579, #6312 ), #22201, .T. ) ;
#18346=DIRECTION ( 'NONE',  ( 0.000000000000000000, 1.000000000000000000, 0.000000000000000000 ) ) ;
#18350=CIRCLE ( 'NONE', #20620, 0.6212598425196850238 ) ;
#18353=B_SPLINE_CURVE_WITH_KNOTS ( 'NONE', 3,
 ( #7310, #13521, #424, #26800, #13811, #22016 ),
 .UNSPECIFIED., .F., .F.,
 ( 4, 2, 4 ),
 ( 0.3108507187342950395, 0.3125269569790670166, 0.3142031952238389936 ),
 .UNSPECIFIED. ) ;
#18356=VERTEX_POINT ( 'NONE', #14943 ) ;
#18360=CARTESIAN_POINT ( 'NONE',  ( -0.6241612306976536129, 0.1093779649445508623, 0.1061598535652353986 ) ) ;
#18370=DIRECTION ( 'NONE',  ( 1.224646799147353207E-16, 1.000000000000000000, -0.000000000000000000 ) ) ;
#18397=FACE_OUTER_BOUND ( 'NONE', #6502, .T. ) ;
#18404=CIRCLE ( 'NONE', #27471, 0.6212598425196850238 ) ;
#18435=FACE_OUTER_BOUND ( 'NONE', #11649, .T. ) ;
#18446=FACE_OUTER_BOUND ( 'NONE', #17769, .T. ) ;
#18456=CARTESIAN_POINT ( 'NONE',  ( 0.1580799066051610802, -0.4326553680327476781, 0.1639447408217406810 ) ) ;
#18472=DIRECTION ( 'NONE',  ( 0.000000000000000000, 1.000000000000000000, 0.000000000000000000 ) ) ;
#18480=EDGE_CURVE ( 'NONE', #8098, #730, #19795, .T. ) ;
#18485=CARTESIAN_POINT ( 'NONE',  ( 0.3937007874015748254, 0.000000000000000000, 0.3425196850393700809 ) ) ;
#18489=ORIENTED_EDGE ( 'NONE', *, *, #14386, .F. ) ;
#18490=CARTESIAN_POINT ( 'NONE',  ( 0.2973550541877014175, 0.3552623538112074097, 0.1494804571810765259 ) ) ;
#18494=DIRECTION ( 'NONE',  ( 0.000000000000000000, 1.000000000000000000, 0.000000000000000000 ) ) ;
#18495=FACE_OUTER_BOUND ( 'NONE', #21198, .T. ) ;
#18509=CARTESIAN_POINT ( 'NONE',  ( -0.4932821129636645874, 0.08637579872942342807, 0.2574803149606298969 ) ) ;
#18517=ORIENTED_EDGE ( 'NONE', *, *, #12576, .F. ) ;
#18536=CARTESIAN_POINT ( 'NONE',  ( 0.000000000000000000, 0.000000000000000000, 0.1771653543307086520 ) ) ;
#18542=ORIENTED_EDGE ( 'NONE', *, *, #15878, .F. ) ;
#18568=ORIENTED_EDGE ( 'NONE', *, *, #25423, .F. ) ;
#18569=ORIENTED_EDGE ( 'NONE', *, *, #19919, .T. ) ;
#18571=FACE_OUTER_BOUND ( 'NONE', #12329, .T. ) ;
#18606=VERTEX_POINT ( 'NONE', #7051 ) ;
#18610=ORIENTED_EDGE ( 'NONE', *, *, #17818, .T. ) ;
#18612=EDGE_CURVE ( 'NONE', #25825, #11779, #20256, .T. ) ;
#18624=CARTESIAN_POINT ( 'NONE',  ( 0.2118615749922956593, -0.5840192333899354438, 0.09685039370078740717 ) ) ;
#18637=EDGE_CURVE ( 'NONE', #20701, #20032, #15351, .T. ) ;
#18660=CARTESIAN_POINT ( 'NONE',  ( 0.5525004126151165096, 0.09742072959660433296, 0.07676968503937006694 ) ) ;
#18666=CARTESIAN_POINT ( 'NONE',  ( 0.4055118110236220486, 0.000000000000000000, 0.3425196850393700809 ) ) ;
#18678=CARTESIAN_POINT ( 'NONE',  ( 0.000000000000000000, 0.000000000000000000, 0.01181102362204724393 ) ) ;
#18683=DIRECTION ( 'NONE',  ( -0.7660444431189774583, 0.6427876096865400291, 0.000000000000000000 ) ) ;
#18689=CIRCLE ( 'NONE', #26356, 0.1003956692913385573 ) ;
#18697=ORIENTED_EDGE ( 'NONE', *, *, #4467, .T. ) ;
#18705=FILL_AREA_STYLE ('',( #20977 ) ) ;
#18706=EDGE_LOOP ( 'NONE', ( #12171, #15304, #6241, #12218, #19352 ) ) ;
#18745=ORIENTED_EDGE ( 'NONE', *, *, #4412, .T. ) ;
#18759=ORIENTED_EDGE ( 'NONE', *, *, #588, .F. ) ;
#18762=CARTESIAN_POINT ( 'NONE',  ( 0.5382469622846938195, -0.3102483656526054956, 0.09684874924366436433 ) ) ;
#18764=ORIENTED_EDGE ( 'NONE', *, *, #765, .T. ) ;
#18765=CARTESIAN_POINT ( 'NONE',  ( -0.3220512119205936608, 0.3834984712787528061, 0.2574827755769819038 ) ) ;
#18774=CARTESIAN_POINT ( 'NONE',  ( -6.132876883919029269E-17, -0.5007874015748031704, 0.04842519685039370358 ) ) ;
#18782=ORIENTED_EDGE ( 'NONE', *, *, #22804, .F. ) ;
#18793=CARTESIAN_POINT ( 'NONE',  ( -0.6342142812989975953, 0.1111449751019639998, 0.2359405056180666482 ) ) ;
#18815=DIRECTION ( 'NONE',  ( 1.000000000000000000, 0.000000000000000000, 0.000000000000000000 ) ) ;
#18822=CARTESIAN_POINT ( 'NONE',  ( 0.000000000000000000, 0.000000000000000000, 0.3543307086614173040 ) ) ;
#18841=CYLINDRICAL_SURFACE ( 'NONE', #24219, 0.6212598425196850238 ) ;
#18846=CARTESIAN_POINT ( 'NONE',  ( 0.2208527687086046520, -0.6048181665998788592, 0.2359405056165906622 ) ) ;
#18853=CARTESIAN_POINT ( 'NONE',  ( 0.5007874015748031704, 0.000000000000000000, 0.2574803149606298969 ) ) ;
#18855=FACE_BOUND ( 'NONE', #7788, .T. ) ;
#18857=VERTEX_POINT ( 'NONE', #26736 ) ;
#18870=CARTESIAN_POINT ( 'NONE',  ( 0.0006832381873102289253, 0.6614169699453786855, 0.1616495878897075689 ) ) ;
#18873=CARTESIAN_POINT ( 'NONE',  ( -0.0005939837304750000086, 0.5007870493127504208, 0.09685039370078740717 ) ) ;
#18881=ORIENTED_EDGE ( 'NONE', *, *, #2646, .T. ) ;
#18882=VERTEX_POINT ( 'NONE', #16299 ) ;
#18887=CARTESIAN_POINT ( 'NONE',  ( -0.4143937130615245046, 0.4928070724629356469, 0.2359405056176802906 ) ) ;
#18902=CARTESIAN_POINT ( 'NONE',  ( 0.1707210962531913734, -0.4707890492249701131, 0.2574803149606298969 ) ) ;
#18912=EDGE_CURVE ( 'NONE', #24718, #9254, #19877, .T. ) ;
#18917=DIRECTION ( 'NONE',  ( 0.000000000000000000, 0.000000000000000000, 1.000000000000000000 ) ) ;
#18944=ORIENTED_EDGE ( 'NONE', *, *, #21767, .F. ) ;
#18957=B_SPLINE_CURVE_WITH_KNOTS ( 'NONE', 3,
 ( #3511, #25282, #18306, #5481, #9848, #27375 ),
 .UNSPECIFIED., .F., .F.,
 ( 4, 2, 4 ),
 ( 0.5000000000000000000, 0.7500000000000000000, 1.000000000000000000 ),
 .UNSPECIFIED. ) ;
#18967=EDGE_CURVE ( 'NONE', #14646, #13130, #10671, .T. ) ;
#18970=FACE_OUTER_BOUND ( 'NONE', #4918, .T. ) ;
#18972=CYLINDRICAL_SURFACE ( 'NONE', #1871, 0.5007874015748031704 ) ;
#18976=TOROIDAL_SURFACE ( 'NONE', #6352, 0.5610236220472440971, 0.1003937007874015908 ) ;
#18996=B_SPLINE_CURVE_WITH_KNOTS ( 'NONE', 3,
 ( #23577, #1525, #5918, #3783, #12404, #21018, #10272, #18887, #16784, #25397 ),
 .UNSPECIFIED., .F., .F.,
 ( 4, 2, 2, 2, 4 ),
 ( 0.000000000000000000, 0.2500000000000000000, 0.5000000000000000000, 0.7500000000000000000, 1.000000000000000000 ),
 .UNSPECIFIED. ) ;
#18999=EDGE_LOOP ( 'NONE', ( #18944, #17212, #22404, #19899 ) ) ;
#19017=AXIS2_PLACEMENT_3D ( 'NONE', #17025, #1345, #12076 ) ;
#19028=AXIS2_PLACEMENT_3D ( 'NONE', #5822, #14747, #23353 ) ;
#19044=CARTESIAN_POINT ( 'NONE',  ( 0.2128972891168661452, -0.5836425148029424914, 0.09684874924366436433 ) ) ;
#19054=AXIS2_PLACEMENT_3D ( 'NONE', #4864, #19721, #9230 ) ;
#19057=CARTESIAN_POINT ( 'NONE',  ( -0.4930758245789425009, 0.08754571829529331217, 0.09685039370078740717 ) ) ;
#19065=DIRECTION ( 'NONE',  ( 0.000000000000000000, -1.000000000000000000, 0.000000000000000000 ) ) ;
#19070=CARTESIAN_POINT ( 'NONE',  ( 0.4932821129636645874, 0.08637579872942321990, 0.09685039370078740717 ) ) ;
#19071=CARTESIAN_POINT ( 'NONE',  ( 0.5525004126151165096, 0.09742072959660433296, 0.1771653543307086520 ) ) ;
#19079=CARTESIAN_POINT ( 'NONE',  ( -0.4537304931026617250, 0.07942646906834199827, 0.1903859677797853645 ) ) ;
#19082=FACE_OUTER_BOUND ( 'NONE', #18706, .T. ) ;
#19086=CARTESIAN_POINT ( 'NONE',  ( 0.0005855335178306408407, 0.4865383137630506782, 0.2467937632983550900 ) ) ;
#19109=ORIENTED_EDGE ( 'NONE', *, *, #23992, .T. ) ;
#19111=CARTESIAN_POINT ( 'NONE',  ( 0.000000000000000000, 0.000000000000000000, 0.1771653543307086520 ) ) ;
#19117=ORIENTED_EDGE ( 'NONE', *, *, #12287, .F. ) ;
#19130=CARTESIAN_POINT ( 'NONE',  ( 0.3995066426835732765, 0.4757712504659606378, 0.09684793308443542803 ) ) ;
#19151=CARTESIAN_POINT ( 'NONE',  ( 0.4333973147258542991, -0.2509079296564015737, 0.2574803149606298969 ) ) ;
#19155=DIRECTION ( 'NONE',  ( 0.000000000000000000, -1.000000000000000000, 0.000000000000000000 ) ) ;
#19163=ADVANCED_FACE ( 'NONE', ( #26260 ), #753, .T. ) ;
#19169=ORIENTED_EDGE ( 'NONE', *, *, #15471, .F. ) ;
#19174=CARTESIAN_POINT ( 'NONE',  ( 0.4688657571997049134, 0.08326155277540096822, 0.2330651858139422827 ) ) ;
#19186=EDGE_LOOP ( 'NONE', ( #17771, #27731, #9019, #19109, #14635 ) ) ;
#19198=AXIS2_PLACEMENT_3D ( 'NONE', #6981, #26586, #22081 ) ;
#19204=EDGE_CURVE ( 'NONE', #27489, #17779, #21232, .T. ) ;
#19210=DIRECTION ( 'NONE',  ( 0.000000000000000000, 0.000000000000000000, 1.000000000000000000 ) ) ;
#19212=ORIENTED_EDGE ( 'NONE', *, *, #3828, .F. ) ;
#19218=EDGE_CURVE ( 'NONE', #13130, #1165, #24649, .T. ) ;
#19226=ORIENTED_EDGE ( 'NONE', *, *, #26451, .T. ) ;
#19227=CARTESIAN_POINT ( 'NONE',  ( 0.000000000000000000, 0.000000000000000000, 0.3425196850393700809 ) ) ;
#19228=CARTESIAN_POINT ( 'NONE',  ( 0.5376957092749645728, -0.3112026930392428614, 0.09685039370078740717 ) ) ;
#19251=DIRECTION ( 'NONE',  ( 0.000000000000000000, 0.000000000000000000, 1.000000000000000000 ) ) ;
#19253=DIRECTION ( 'NONE',  ( 0.000000000000000000, 0.000000000000000000, 1.000000000000000000 ) ) ;
#19258=CARTESIAN_POINT ( 'NONE',  ( -0.4338922498494567348, -0.2500511477696472085, 0.2574819596263889787 ) ) ;
#19310=DIRECTION ( 'NONE',  ( 1.000000000000000000, 0.000000000000000000, 0.000000000000000000 ) ) ;
#19313=ORIENTED_EDGE ( 'NONE', *, *, #9757, .F. ) ;
#19332=CARTESIAN_POINT ( 'NONE',  ( 0.4015002836602225567, -0.2311469024248521409, 0.2048502514551664710 ) ) ;
#19335=B_SPLINE_CURVE_WITH_KNOTS ( 'NONE', 3,
 ( #26033, #4819, #4288, #2691, #12894, #15037 ),
 .UNSPECIFIED., .F., .F.,
 ( 4, 2, 4 ),
 ( 0.5000000000000000000, 0.7500000000000000000, 1.000000000000000000 ),
 .UNSPECIFIED. ) ;
#19352=ORIENTED_EDGE ( 'NONE', *, *, #18637, .T. ) ;
#19367=DIRECTION ( 'NONE',  ( 0.6427876096865398070, 0.7660444431189775694, -0.000000000000000000 ) ) ;
#19368=EDGE_CURVE ( 'NONE', #4739, #5673, #22364, .T. ) ;
#19391=ORIENTED_EDGE ( 'NONE', *, *, #15524, .T. ) ;
#19399=DIRECTION ( 'NONE',  ( 1.000000000000000000, 0.000000000000000000, 0.000000000000000000 ) ) ;
#19404=VERTEX_POINT ( 'NONE', #26949 ) ;
#19405=DIRECTION ( 'NONE',  ( 0.000000000000000000, 0.000000000000000000, 1.000000000000000000 ) ) ;
#19411=CARTESIAN_POINT ( 'NONE',  ( 0.000000000000000000, 0.000000000000000000, 0.2574803149606298969 ) ) ;
#19421=CARTESIAN_POINT ( 'NONE',  ( 0.2173565190923199553, -0.5952284643130145714, 0.1061598535646071789 ) ) ;
#19436=CARTESIAN_POINT ( 'NONE',  ( 0.000000000000000000, 0.5610236220472440971, 0.1771653543307086520 ) ) ;
#19437=CIRCLE ( 'NONE', #2290, 0.5007874015748031704 ) ;
#19442=ORIENTED_EDGE ( 'NONE', *, *, #24754, .T. ) ;
#19468=CARTESIAN_POINT ( 'NONE',  ( 0.000000000000000000, 0.000000000000000000, 0.09685039370078740717 ) ) ;
#19469=DIRECTION ( 'NONE',  ( 0.000000000000000000, 0.000000000000000000, 1.000000000000000000 ) ) ;
#19470=CARTESIAN_POINT ( 'NONE',  ( 0.3992017438595157897, -0.2298214351608010297, 0.1903859677804414230 ) ) ;
#19473=CARTESIAN_POINT ( 'NONE',  ( -0.1570092758121678089, -0.4330450457732858416, 0.1771653543307084855 ) ) ;
#19505=CIRCLE ( 'NONE', #23127, 0.1003956692913385851 ) ;
#19510=CARTESIAN_POINT ( 'NONE',  ( -7.608238775805210269E-17, -0.6212598425196850238, 0.3543307086614173040 ) ) ;
#19514=B_SPLINE_CURVE_WITH_KNOTS ( 'NONE', 3,
 ( #15205, #8691, #6578, #19575, #23949, #4585 ),
 .UNSPECIFIED., .F., .F.,
 ( 4, 2, 4 ),
 ( 0.000000000000000000, 0.2500000000000000000, 0.5000000000000000000 ),
 .UNSPECIFIED. ) ;
#19540=AXIS2_PLACEMENT_3D ( 'NONE', #4245, #19210, #19065 ) ;
#19550=APPLICATION_CONTEXT ( 'automotive_design' ) ;
#19553=DIRECTION ( 'NONE',  ( 0.6427876096865396960, 0.7660444431189776804, -0.000000000000000000 ) ) ;
#19560=VERTEX_POINT ( 'NONE', #23401 ) ;
#19575=CARTESIAN_POINT ( 'NONE',  ( -0.4015002836661830110, -0.2311469024283132612, 0.1494804571819171590 ) ) ;
#19576=CIRCLE ( 'NONE', #11876, 0.4606299212598425341 ) ;
#19582=CARTESIAN_POINT ( 'NONE',  ( 0.2965233727166234345, 0.3524965443697388179, 0.1639447408612718093 ) ) ;
#19606=CARTESIAN_POINT ( 'NONE',  ( -0.3223547283257516272, 0.3832433309296771617, 0.2574803149606298969 ) ) ;
#19616=DIRECTION ( 'NONE',  ( 0.000000000000000000, 0.000000000000000000, 1.000000000000000000 ) ) ;
#19626=DIRECTION ( 'NONE',  ( 0.000000000000000000, 0.000000000000000000, 1.000000000000000000 ) ) ;
#19635=ORIENTED_EDGE ( 'NONE', *, *, #705, .F. ) ;
#19654=EDGE_CURVE ( 'NONE', #16979, #2747, #14493, .T. ) ;
#19658=CARTESIAN_POINT ( 'NONE',  ( 0.5572789388089177676, -0.3225230913470072402, 0.2359405056200655770 ) ) ;
#19674=ORIENTED_EDGE ( 'NONE', *, *, #15636, .F. ) ;
#19686=EDGE_CURVE ( 'NONE', #6596, #1165, #17832, .T. ) ;
#19694=EDGE_CURVE ( 'NONE', #6066, #14064, #5667, .T. ) ;
#19716=DIRECTION ( 'NONE',  ( 0.7660444431189780135, 0.6427876096865392519, 0.000000000000000000 ) ) ;
#19720=ORIENTED_EDGE ( 'NONE', *, *, #26796, .T. ) ;
#19721=DIRECTION ( 'NONE',  ( 0.000000000000000000, -1.000000000000000000, 0.000000000000000000 ) ) ;
#19730=EDGE_LOOP ( 'NONE', ( #20706, #9726, #7430, #5789 ) ) ;
#19731=CARTESIAN_POINT ( 'NONE',  ( -0.6117062799105531523, 0.1085321106658068829, 0.2574803149606298969 ) ) ;
#19743=CARTESIAN_POINT ( 'NONE',  ( -0.3606190329934327310, 0.4297690281277732338, 0.07676968503937006694 ) ) ;
#19744=AXIS2_PLACEMENT_3D ( 'NONE', #13576, #2823, #11464 ) ;
#19763=CARTESIAN_POINT ( 'NONE',  ( -0.3122922550262028363, 0.3730863453119290241, 0.2467937632973297712 ) ) ;
#19767=DIRECTION ( 'NONE',  ( 0.000000000000000000, -1.000000000000000000, 0.000000000000000000 ) ) ;
#19777=CARTESIAN_POINT ( 'NONE',  ( 0.2956505864974371400, 0.3532288989643546651, 0.1771653543307085410 ) ) ;
#19785=CARTESIAN_POINT ( 'NONE',  ( 0.5484420430263082791, -0.3174147232942853836, 0.1061598535660860931 ) ) ;
#19787=CARTESIAN_POINT ( 'NONE',  ( -0.4858607088160732390, -0.2805118110236220486, 0.1771653543307086520 ) ) ;
#19795=CIRCLE ( 'NONE', #7626, 0.3937007874015748254 ) ;
#19797=EDGE_CURVE ( 'NONE', #26549, #17148, #5703, .T. ) ;
#19826=EDGE_CURVE ( 'NONE', #11359, #9393, #23327, .T. ) ;
#19828=EDGE_CURVE ( 'NONE', #6574, #13188, #14184, .T. ) ;
#19834=CYLINDRICAL_SURFACE ( 'NONE', #27203, 0.6212598425196850238 ) ;
#19845=ADVANCED_FACE ( 'NONE', ( #5557, #625 ), #16013, .T. ) ;
#19846=B_SPLINE_CURVE_WITH_KNOTS ( 'NONE', 3,
 ( #26985, #12285, #13993, #9885, #1551, #10025 ),
 .UNSPECIFIED., .F., .F.,
 ( 4, 2, 4 ),
 ( 0.9359046326922999537, 0.9375808709372039917, 0.9392571091821070306 ),
 .UNSPECIFIED. ) ;
#19871=ADVANCED_FACE ( 'NONE', ( #24898, #3273 ), #26590, .T. ) ;
#19877=B_SPLINE_CURVE_WITH_KNOTS ( 'NONE', 3,
 ( #40, #25841, #6490, #8741 ),
 .UNSPECIFIED., .F., .F.,
 ( 4, 4 ),
 ( 0.9375808709372031036, 0.9392571091818440188 ),
 .UNSPECIFIED. ) ;
#19880=ORIENTED_EDGE ( 'NONE', *, *, #4448, .F. ) ;
#19893=CARTESIAN_POINT ( 'NONE',  ( -0.2122766679520244337, -0.5838685267775873822, 0.09684793308443542803 ) ) ;
#19894=CARTESIAN_POINT ( 'NONE',  ( 0.000000000000000000, 0.000000000000000000, 0.2574803149606298969 ) ) ;
#19899=ORIENTED_EDGE ( 'NONE', *, *, #2070, .T. ) ;
#19901=SHAPE_REPRESENTATION_RELATIONSHIP ( 'NONE' , 'NONE' ,  #1615, #8670 ) ;
#19904=ORIENTED_EDGE ( 'NONE', *, *, #22815, .F. ) ;
#19906=CIRCLE ( 'NONE', #27135, 0.6212598425196850238 ) ;
#19909=EDGE_LOOP ( 'NONE', ( #27174, #24838, #21477, #1739 ) ) ;
#19919=EDGE_CURVE ( 'NONE', #2920, #730, #25088, .T. ) ;
#19928=DIRECTION ( 'NONE',  ( 0.000000000000000000, 0.000000000000000000, 1.000000000000000000 ) ) ;
#19930=CARTESIAN_POINT ( 'NONE',  ( -0.4339912984563299436, -0.2498791196563492356, 0.2574803149606298969 ) ) ;
#19931=B_SPLINE_CURVE_WITH_KNOTS ( 'NONE', 3,
 ( #3802, #14980, #6483, #19332, #19470, #2232 ),
 .UNSPECIFIED., .F., .F.,
 ( 4, 2, 4 ),
 ( 0.000000000000000000, 0.2500000000000000000, 0.5000000000000000000 ),
 .UNSPECIFIED. ) ;
#19935=DIRECTION ( 'NONE',  ( 1.224646799147353207E-16, 1.000000000000000000, -0.000000000000000000 ) ) ;
#19941=DIRECTION ( 'NONE',  ( 0.000000000000000000, 0.000000000000000000, 1.000000000000000000 ) ) ;
#19967=CARTESIAN_POINT ( 'NONE',  ( -0.0006812437162536292114, 0.6577569867595576270, 0.1461456498329627707 ) ) ;
#19990=CARTESIAN_POINT ( 'NONE',  ( -0.0004405150045524263542, 0.6212597256746514862, 0.2574819594177531479 ) ) ;
#19992=ORIENTED_EDGE ( 'NONE', *, *, #6732, .F. ) ;
#20011=CARTESIAN_POINT ( 'NONE',  ( -0.3214446924536846772, 0.3840069416942866742, 0.09685039370078740717 ) ) ;
#20015=DIRECTION ( 'NONE',  ( 1.000000000000000000, 0.000000000000000000, 0.000000000000000000 ) ) ;
#20032=VERTEX_POINT ( 'NONE', #5706 ) ;
#20060=DIRECTION ( 'NONE',  ( 0.000000000000000000, 0.000000000000000000, 1.000000000000000000 ) ) ;
#20070=CARTESIAN_POINT ( 'NONE',  ( -0.4537304931026616139, 0.07942646906834205378, 0.1771653543307086243 ) ) ;
#20080=CIRCLE ( 'NONE', #7917, 0.5007874015748031704 ) ;
#20099=CARTESIAN_POINT ( 'NONE',  ( 0.4143937130606526464, 0.4928070724618983101, 0.2359405056194269767 ) ) ;
#20103=DIRECTION ( 'NONE',  ( -0.5000000000000002220, -0.8660254037844384856, 0.000000000000000000 ) ) ;
#20111=CARTESIAN_POINT ( 'NONE',  ( -0.4932478747986535628, 0.08657132889677658649, 0.09684874903502814492 ) ) ;
#20131=B_SPLINE_CURVE_WITH_KNOTS ( 'NONE', 3,
 ( #24130, #547, #24262, #9143, #4911, #13523 ),
 .UNSPECIFIED., .F., .F.,
 ( 4, 2, 4 ),
 ( 0.000000000000000000, 0.2500000000000000000, 0.5000000000000000000 ),
 .UNSPECIFIED. ) ;
#20148=ORIENTED_EDGE ( 'NONE', *, *, #1101, .F. ) ;
#20158=DIRECTION ( 'NONE',  ( -0.4999999999999997780, -0.8660254037844388186, 0.000000000000000000 ) ) ;
#20160=CARTESIAN_POINT ( 'NONE',  ( 0.3222028160008074682, 0.3833711078595924970, 0.09684874903502814492 ) ) ;
#20169=EDGE_LOOP ( 'NONE', ( #11746, #180, #8557, #7385 ) ) ;
#20199=CARTESIAN_POINT ( 'NONE',  ( 0.4015002836606120229, -0.2311469024250759063, 0.1494804572046649349 ) ) ;
#20201=DIRECTION ( 'NONE',  ( 0.3420201433256691570, 0.9396926207859084279, -0.000000000000000000 ) ) ;
#20218=AXIS2_PLACEMENT_3D ( 'NONE', #22352, #11611, #22495 ) ;
#20226=CIRCLE ( 'NONE', #24713, 0.5007874015748031704 ) ;
#20241=CARTESIAN_POINT ( 'NONE',  ( 0.3220512119205940493, 0.3834984712787528061, 0.2574827755769819038 ) ) ;
#20253=CARTESIAN_POINT ( 'NONE',  ( 0.000000000000000000, 0.000000000000000000, 0.1771653543307086520 ) ) ;
#20256=CIRCLE ( 'NONE', #20275, 0.5007874015748031704 ) ;
#20262=TOROIDAL_SURFACE ( 'NONE', #10791, 0.5610236220472440971, 0.1003937007874015908 ) ;
#20265=VERTEX_POINT ( 'NONE', #27878 ) ;
#20270=ORIENTED_EDGE ( 'NONE', *, *, #15822, .T. ) ;
#20275=AXIS2_PLACEMENT_3D ( 'NONE', #6644, #15272, #23882 ) ;
#20284=VERTEX_POINT ( 'NONE', #12884 ) ;
#20289=ORIENTED_EDGE ( 'NONE', *, *, #25423, .T. ) ;
#20303=CARTESIAN_POINT ( 'NONE',  ( 0.4930758245789425009, 0.08754571829529310401, 0.09685039370078740717 ) ) ;
#20308=DIRECTION ( 'NONE',  ( 0.1736481776669313581, 0.9848077530122080203, 0.000000000000000000 ) ) ;
#20335=DIRECTION ( 'NONE',  ( 0.000000000000000000, 0.000000000000000000, 1.000000000000000000 ) ) ;
#20342=ORIENTED_EDGE ( 'NONE', *, *, #21703, .F. ) ;
#20350=ORIENTED_EDGE ( 'NONE', *, *, #26796, .F. ) ;
#20354=EDGE_CURVE ( 'NONE', #1869, #27489, #16168, .T. ) ;
#20360=CARTESIAN_POINT ( 'NONE',  ( 0.4333973147258542991, -0.2509079296564015737, 0.2574803149606298969 ) ) ;
#20372=FACE_OUTER_BOUND ( 'NONE', #5029, .T. ) ;
#20377=EDGE_CURVE ( 'NONE', #6124, #7423, #20226, .T. ) ;
#20399=CARTESIAN_POINT ( 'NONE',  ( 0.000000000000000000, 0.7283464566929134243, 0.1771653543307086520 ) ) ;
#20400=CARTESIAN_POINT ( 'NONE',  ( 0.1918813796216842782, -0.5271897577243779276, 0.2775610236220472093 ) ) ;
#20432=SPHERICAL_SURFACE ( 'NONE', #3612, 0.1003956692913385851 ) ;
#20437=AXIS2_PLACEMENT_3D ( 'NONE', #21050, #16680, #4106 ) ;
#20446=CARTESIAN_POINT ( 'NONE',  ( 0.3215969074633125979, 0.3838795254899315390, 0.09684874903502814492 ) ) ;
#20447=SPHERICAL_SURFACE ( 'NONE', #8078, 0.1003956692913385851 ) ;
#20464=AXIS2_PLACEMENT_3D ( 'NONE', #3670, #10166, #8354 ) ;
#20466=CARTESIAN_POINT ( 'NONE',  ( 0.4335958738490826581, -0.2505647196907697105, 0.09684793308443523374 ) ) ;
#20467=ORIENTED_EDGE ( 'NONE', *, *, #25561, .F. ) ;
#20469=CIRCLE ( 'NONE', #8302, 0.6212598425196850238 ) ;
#20500=ADVANCED_FACE ( 'NONE', ( #18495 ), #23400, .T. ) ;
#20502=FACE_OUTER_BOUND ( 'NONE', #19730, .T. ) ;
#20518=ORIENTED_EDGE ( 'NONE', *, *, #26119, .T. ) ;
#20526=CARTESIAN_POINT ( 'NONE',  ( 0.4256740239334655951, 0.5062356173693111083, 0.1616495878840815137 ) ) ;
#20533=VERTEX_POINT ( 'NONE', #10165 ) ;
#20574=AXIS2_PLACEMENT_3D ( 'NONE', #12019, #9894, #18494 ) ;
#20588=DIRECTION ( 'NONE',  ( 1.000000000000000000, 0.000000000000000000, 0.000000000000000000 ) ) ;
#20594=FACE_OUTER_BOUND ( 'NONE', #23842, .T. ) ;
#20603=DIRECTION ( 'NONE',  ( 0.000000000000000000, 0.000000000000000000, -1.000000000000000000 ) ) ;
#20613=TOROIDAL_SURFACE ( 'NONE', #8434, 0.5610236220472440971, 0.1003937007874015908 ) ;
#20620=AXIS2_PLACEMENT_3D ( 'NONE', #21120, #10095, #8128 ) ;
#20640=CARTESIAN_POINT ( 'NONE',  ( -0.3223547283257516272, 0.3832433309296771617, 0.2574803149606298969 ) ) ;
#20650=CARTESIAN_POINT ( 'NONE',  ( 0.6212598425196851348, 0.000000000000000000, 0.09685039370078740717 ) ) ;
#20660=CARTESIAN_POINT ( 'NONE',  ( 0.000000000000000000, 0.7283464566929134243, 0.3425196850393700809 ) ) ;
#20663=CIRCLE ( 'NONE', #7576, 0.1003956692913385851 ) ;
#20673=ORIENTED_EDGE ( 'NONE', *, *, #19368, .T. ) ;
#20675=CARTESIAN_POINT ( 'NONE',  ( -0.4931450244001936989, 0.08715529520342381320, 0.09684793308443542803 ) ) ;
#20693=ORIENTED_EDGE ( 'NONE', *, *, #6586, .F. ) ;
#20700=SURFACE_STYLE_USAGE ( .BOTH. , #25502 ) ;
#20701=VERTEX_POINT ( 'NONE', #26130 ) ;
#20703=EDGE_CURVE ( 'NONE', #14659, #17723, #23879, .T. ) ;
#20706=ORIENTED_EDGE ( 'NONE', *, *, #17447, .T. ) ;
#20711=VERTEX_POINT ( 'NONE', #6367 ) ;
#20715=SPHERICAL_SURFACE ( 'NONE', #20784, 0.1003956692913385851 ) ;
#20721=B_SPLINE_CURVE_WITH_KNOTS ( 'NONE', 3,
 ( #16073, #15792, #7740, #18156, #16354, #24956 ),
 .UNSPECIFIED., .F., .F.,
 ( 4, 2, 4 ),
 ( 0.9359046326922999537, 0.9375808709372039917, 0.9392571091821070306 ),
 .UNSPECIFIED. ) ;
#20726=AXIS2_PLACEMENT_3D ( 'NONE', #24145, #20603, #7755 ) ;
#20730=CARTESIAN_POINT ( 'NONE',  ( -0.4535326485287287657, 0.08054850140359764987, 0.1771653543307088186 ) ) ;
#20751=AXIS2_PLACEMENT_3D ( 'NONE', #3601, #18178, #5751 ) ;
#20756=DIRECTION ( 'NONE',  ( 0.000000000000000000, 0.000000000000000000, 1.000000000000000000 ) ) ;
#20757=CARTESIAN_POINT ( 'NONE',  ( 0.000000000000000000, 0.000000000000000000, 0.1771653543307086520 ) ) ;
#20761=DIRECTION ( 'NONE',  ( 0.000000000000000000, 0.000000000000000000, 1.000000000000000000 ) ) ;
#20770=CIRCLE ( 'NONE', #26616, 0.6212598425196850238 ) ;
#20771=ORIENTED_EDGE ( 'NONE', *, *, #27512, .F. ) ;
#20784=AXIS2_PLACEMENT_3D ( 'NONE', #1360, #27215, #23125 ) ;
#20787=CARTESIAN_POINT ( 'NONE',  ( -0.6342142812942709318, 0.1111449751011379800, 0.1183902030371653535 ) ) ;
#20799=DIRECTION ( 'NONE',  ( 1.000000000000000000, 0.000000000000000000, 0.000000000000000000 ) ) ;
#20802=AXIS2_PLACEMENT_3D ( 'NONE', #2057, #25652, #6310 ) ;
#20810=CARTESIAN_POINT ( 'NONE',  ( 0.4339912984563291110, -0.2498791196563492356, 0.2574803149606298969 ) ) ;
#20826=AXIS2_PLACEMENT_3D ( 'NONE', #18084, #9632, #7528 ) ;
#20833=CARTESIAN_POINT ( 'NONE',  ( 0.3991696156513551141, 0.4760540497243913594, 0.09684793308443542803 ) ) ;
#20850=CARTESIAN_POINT ( 'NONE',  ( 0.000000000000000000, 0.000000000000000000, 0.2574803149606298969 ) ) ;
#20870=PRODUCT_CONTEXT ( 'NONE', #19550, 'mechanical' ) ;
#20878=ORIENTED_EDGE ( 'NONE', *, *, #2419, .F. ) ;
#20895=CARTESIAN_POINT ( 'NONE',  ( 0.0006615832605804723319, 0.6212594902576319411, 0.2574803149606298969 ) ) ;
#20908=DIRECTION ( 'NONE',  ( 0.1736481776669313581, 0.9848077530122080203, 0.000000000000000000 ) ) ;
#20911=ORIENTED_EDGE ( 'NONE', *, *, #22305, .F. ) ;
#20916=CARTESIAN_POINT ( 'NONE',  ( -0.6117062799105453808, 0.1085321106658580781, 0.09685039370078740717 ) ) ;
#20920=VERTEX_POINT ( 'NONE', #10948 ) ;
#20928=TOROIDAL_SURFACE ( 'NONE', #6958, 0.4055118110236220486, 0.01181102362204724393 ) ;
#20935=CIRCLE ( 'NONE', #17772, 0.7283464566929134243 ) ;
#20938=DIRECTION ( 'NONE',  ( 0.000000000000000000, 0.000000000000000000, 1.000000000000000000 ) ) ;
#20941=AXIS2_PLACEMENT_3D ( 'NONE', #22147, #4769, #8877 ) ;
#20945=DIRECTION ( 'NONE',  ( 0.000000000000000000, 0.000000000000000000, -1.000000000000000000 ) ) ;
#20962=ORIENTED_EDGE ( 'NONE', *, *, #25470, .T. ) ;
#20977=FILL_AREA_STYLE_COLOUR ( '', #10694 ) ;
#20991=DIRECTION ( 'NONE',  ( 0.000000000000000000, 0.000000000000000000, 1.000000000000000000 ) ) ;
#21001=CARTESIAN_POINT ( 'NONE',  ( 0.000000000000000000, 0.000000000000000000, 0.04842519685039370358 ) ) ;
#21005=AXIS2_PLACEMENT_3D ( 'NONE', #26875, #27028, #24604 ) ;
#21018=CARTESIAN_POINT ( 'NONE',  ( -0.4256740239345673249, 0.5062356173706242801, 0.1926811207662450509 ) ) ;
#21031=CARTESIAN_POINT ( 'NONE',  ( 0.2131049448083992270, -0.5835666837866889667, 0.09685039370078740717 ) ) ;
#21034=ORIENTED_EDGE ( 'NONE', *, *, #4503, .F. ) ;
#21040=AXIS2_PLACEMENT_3D ( 'NONE', #9348, #24610, #1044 ) ;
#21042=LINE ( 'NONE', #18774, #13284 ) ;
#21050=CARTESIAN_POINT ( 'NONE',  ( 0.000000000000000000, 0.000000000000000000, 0.01181102362204724393 ) ) ;
#21055=AXIS2_PLACEMENT_3D ( 'NONE', #7123, #24349, #17584 ) ;
#21064=DIRECTION ( 'NONE',  ( 0.9848077530122080203, -0.1736481776669309973, 0.000000000000000000 ) ) ;
#21073=PRODUCT ( 'Deep Groove Ball Bearing 20x37x9', 'Deep Groove Ball Bearing 20x37x9', '', ( #20870 ) ) ;
#21077=ORIENTED_EDGE ( 'NONE', *, *, #6732, .T. ) ;
#21091=EDGE_LOOP ( 'NONE', ( #15865, #7033, #14950, #18745, #3413, #6226, #15834, #7844, #6707, #21341, #4730, #16723, #5460 ) ) ;
#21108=DIRECTION ( 'NONE',  ( 0.000000000000000000, 0.000000000000000000, 1.000000000000000000 ) ) ;
#21120=CARTESIAN_POINT ( 'NONE',  ( 0.000000000000000000, 0.000000000000000000, 0.09685039370078740717 ) ) ;
#21128=ORIENTED_EDGE ( 'NONE', *, *, #10300, .T. ) ;
#21133=CARTESIAN_POINT ( 'NONE',  ( -0.4932821129636645874, 0.08637579872942342807, 0.09685039370078740717 ) ) ;
#21140=CARTESIAN_POINT ( 'NONE',  ( 1.456051859513969730E-17, 0.5007874015748032814, 0.2574827755769819038 ) ) ;
#21147=CARTESIAN_POINT ( 'NONE',  ( -0.3988311005573134116, 0.4763376377694984454, 0.09685039370078740717 ) ) ;
#21155=CARTESIAN_POINT ( 'NONE',  ( -0.2208527687074414714, -0.6048181665966714249, 0.1183902030404290623 ) ) ;
#21160=ORIENTED_EDGE ( 'NONE', *, *, #4708, .T. ) ;
#21165=CARTESIAN_POINT ( 'NONE',  ( -0.2965233727166468047, 0.3524965443697193335, 0.1771653543307085965 ) ) ;
#21168=ORIENTED_EDGE ( 'NONE', *, *, #22193, .T. ) ;
#21171=CIRCLE ( 'NONE', #21637, 0.4606299212598425341 ) ;
#21178=ORIENTED_EDGE ( 'NONE', *, *, #25236, .F. ) ;
#21183=VERTEX_POINT ( 'NONE', #20810 ) ;
#21184=CARTESIAN_POINT ( 'NONE',  ( -0.3215969074633125979, 0.3838795254899315390, 0.2574819596263889787 ) ) ;
#21185=CIRCLE ( 'NONE', #3980, 0.5007874015748031704 ) ;
#21193=B_SPLINE_CURVE_WITH_KNOTS ( 'NONE', 3,
 ( #27565, #2123, #14870, #10451, #184, #19070 ),
 .UNSPECIFIED., .F., .F.,
 ( 4, 2, 4 ),
 ( 0.3000437156586439613, 0.3015484798814579981, 0.3030532441042709801 ),
 .UNSPECIFIED. ) ;
#21196=ORIENTED_EDGE ( 'NONE', *, *, #4096, .F. ) ;
#21198=EDGE_LOOP ( 'NONE', ( #25060, #13028, #11933, #5663, #10362 ) ) ;
#21204=CARTESIAN_POINT ( 'NONE',  ( 0.000000000000000000, 0.000000000000000000, 0.01181102362204724393 ) ) ;
#21214=ADVANCED_FACE ( 'NONE', ( #6271 ), #23515, .F. ) ;
#21221=CARTESIAN_POINT ( 'NONE',  ( 0.0005696707463077370576, 0.4606295689977898400, 0.1771653543307089018 ) ) ;
#21227=EDGE_LOOP ( 'NONE', ( #8815, #15911 ) ) ;
#21232=B_SPLINE_CURVE_WITH_KNOTS ( 'NONE', 3,
 ( #15135, #12988, #17509, #26128, #21618, #6783 ),
 .UNSPECIFIED., .F., .F.,
 ( 4, 2, 4 ),
 ( 0.000000000000000000, 0.2500000000000000000, 0.5000000000000000000 ),
 .UNSPECIFIED. ) ;
#21239=ORIENTED_EDGE ( 'NONE', *, *, #24840, .F. ) ;
#21244=DIRECTION ( 'NONE',  ( 0.000000000000000000, 1.000000000000000000, 0.000000000000000000 ) ) ;
#21265=ORIENTED_EDGE ( 'NONE', *, *, #3506, .F. ) ;
#21268=AXIS2_PLACEMENT_3D ( 'NONE', #10369, #8264, #16888 ) ;
#21292=CARTESIAN_POINT ( 'NONE',  ( 0.000000000000000000, 0.000000000000000000, 0.1771653543307086520 ) ) ;
#21294=CARTESIAN_POINT ( 'NONE',  ( -0.5525004126151165096, 0.09742072959660473541, 0.07676968503937006694 ) ) ;
#21301=AXIS2_PLACEMENT_3D ( 'NONE', #18678, #9935, #23232 ) ;
#21306=EDGE_LOOP ( 'NONE', ( #27297, #10109, #11870, #2188, #21239 ) ) ;
#21337=EDGE_CURVE ( 'NONE', #6451, #13218, #21171, .T. ) ;
#21341=ORIENTED_EDGE ( 'NONE', *, *, #26746, .T. ) ;
#21347=ORIENTED_EDGE ( 'NONE', *, *, #15441, .T. ) ;
#21358=ORIENTED_EDGE ( 'NONE', *, *, #3152, .F. ) ;
#21374=CARTESIAN_POINT ( 'NONE',  ( -6.132876883919029269E-17, -0.5007874015748031704, 0.09685039370078740717 ) ) ;
#21385=DIRECTION ( 'NONE',  ( 0.000000000000000000, 0.000000000000000000, 1.000000000000000000 ) ) ;
#21397=ORIENTED_EDGE ( 'NONE', *, *, #23182, .F. ) ;
#21408=EDGE_CURVE ( 'NONE', #2747, #21183, #6967, .T. ) ;
#21411=ORIENTED_EDGE ( 'NONE', *, *, #10267, .T. ) ;
#21415=EDGE_CURVE ( 'NONE', #13221, #11845, #8325, .T. ) ;
#21423=DIRECTION ( 'NONE',  ( 0.000000000000000000, -1.000000000000000000, 0.000000000000000000 ) ) ;
#21438=AXIS2_PLACEMENT_3D ( 'NONE', #8031, #16358, #3336 ) ;
#21446=VERTEX_POINT ( 'NONE', #16691 ) ;
#21477=ORIENTED_EDGE ( 'NONE', *, *, #27294, .T. ) ;
#21489=AXIS2_PLACEMENT_3D ( 'NONE', #23046, #9752, #8071 ) ;
#21493=EDGE_CURVE ( 'NONE', #3818, #15551, #22624, .T. ) ;
#21514=EDGE_CURVE ( 'NONE', #22691, #8098, #25587, .T. ) ;
#21528=ORIENTED_EDGE ( 'NONE', *, *, #21983, .F. ) ;
#21536=B_SPLINE_CURVE_WITH_KNOTS ( 'NONE', 3,
 ( #1008, #14289, #24720, #3668, #16683, #25292 ),
 .UNSPECIFIED., .F., .F.,
 ( 4, 2, 4 ),
 ( 0.3000437156586439613, 0.3015484798814569989, 0.3030532441042709801 ),
 .UNSPECIFIED. ) ;
#21539=DIRECTION ( 'NONE',  ( 0.000000000000000000, 1.000000000000000000, 0.000000000000000000 ) ) ;
#21556=ADVANCED_FACE ( 'NONE', ( #12997 ), #130, .F. ) ;
#21565=ORIENTED_EDGE ( 'NONE', *, *, #8978, .F. ) ;
#21576=ORIENTED_EDGE ( 'NONE', *, *, #1280, .F. ) ;
#21577=EDGE_LOOP ( 'NONE', ( #13099, #16558, #15109, #19904 ) ) ;
#21610=TOROIDAL_SURFACE ( 'NONE', #1315, 0.5610236220472440971, 0.1003937007874015908 ) ;
#21618=CARTESIAN_POINT ( 'NONE',  ( -0.1580799066051628565, -0.4326553680327470675, 0.1639447408228894565 ) ) ;
#21636=CARTESIAN_POINT ( 'NONE',  ( 0.5724622793726006353, -0.3313001865994052442, 0.1616495878854405099 ) ) ;
#21637=AXIS2_PLACEMENT_3D ( 'NONE', #26032, #27005, #1015 ) ;
#21638=DIRECTION ( 'NONE',  ( 0.4999999999999997780, -0.8660254037844388186, 0.000000000000000000 ) ) ;
#21648=VERTEX_POINT ( 'NONE', #26399 ) ;
#21649=ORIENTED_EDGE ( 'NONE', *, *, #23182, .T. ) ;
#21651=ORIENTED_EDGE ( 'NONE', *, *, #1132, .F. ) ;
#21653=CARTESIAN_POINT ( 'NONE',  ( -0.4121125639592903012, -0.2386018002122738402, 0.1212655228592417339 ) ) ;
#21660=CARTESIAN_POINT ( 'NONE',  ( 0.4246272423003497609, 0.5071139714522435726, 0.1926811207740559140 ) ) ;
#21663=EDGE_CURVE ( 'NONE', #25476, #1804, #22608, .T. ) ;
#21684=CARTESIAN_POINT ( 'NONE',  ( -0.0006681923949046837848, 0.6336721034123411478, 0.1061598535668189930 ) ) ;
#21685=CARTESIAN_POINT ( 'NONE',  ( -0.1570092758121678089, -0.4330450457732858416, 0.1771653543307084855 ) ) ;
#21703=EDGE_CURVE ( 'NONE', #14646, #5816, #2740, .T. ) ;
#21705=CARTESIAN_POINT ( 'NONE',  ( -0.4055118110236220486, 4.966087413865251393E-17, -1.639108858267716421E-17 ) ) ;
#21716=ORIENTED_EDGE ( 'NONE', *, *, #7551, .F. ) ;
#21729=VERTEX_POINT ( 'NONE', #2667 ) ;
#21751=CARTESIAN_POINT ( 'NONE',  ( -0.2956505864974143805, 0.3532288989643738719, 0.1771653543307089018 ) ) ;
#21762=EDGE_CURVE ( 'NONE', #13221, #13188, #9515, .T. ) ;
#21767=EDGE_CURVE ( 'NONE', #20284, #16979, #12688, .T. ) ;
#21791=VERTEX_POINT ( 'NONE', #4737 ) ;
#21793=CARTESIAN_POINT ( 'NONE',  ( 0.7283464566929135353, 0.000000000000000000, 0.01181102362204724393 ) ) ;
#21794=DIRECTION ( 'NONE',  ( 0.000000000000000000, 0.000000000000000000, 1.000000000000000000 ) ) ;
#21814=AXIS2_PLACEMENT_3D ( 'NONE', #25942, #22212, #6595 ) ;
#21822=ORIENTED_EDGE ( 'NONE', *, *, #21493, .F. ) ;
#21824=EDGE_LOOP ( 'NONE', ( #16656, #24248 ) ) ;
#21845=EDGE_LOOP ( 'NONE', ( #1795, #8459, #15165, #23700, #4252, #20693 ) ) ;
#21853=ORIENTED_EDGE ( 'NONE', *, *, #3828, .T. ) ;
#21865=ORIENTED_EDGE ( 'NONE', *, *, #17812, .T. ) ;
#21882=DIRECTION ( 'NONE',  ( 0.000000000000000000, 0.000000000000000000, 1.000000000000000000 ) ) ;
#21886=ORIENTED_EDGE ( 'NONE', *, *, #5056, .F. ) ;
#21902=ORIENTED_EDGE ( 'NONE', *, *, #233, .F. ) ;
#21919=DIRECTION ( 'NONE',  ( 1.000000000000000000, 0.000000000000000000, 0.000000000000000000 ) ) ;
#21929=AXIS2_PLACEMENT_3D ( 'NONE', #13283, #9297, #448 ) ;
#21955=EDGE_CURVE ( 'NONE', #3160, #21729, #7599, .T. ) ;
#21960=CARTESIAN_POINT ( 'NONE',  ( -0.1623262587462485640, -0.4476804331104035084, 0.2330651858513022867 ) ) ;
#21968=CARTESIAN_POINT ( 'NONE',  ( 0.0005789383928823483780, 0.4762008496965042803, 0.1212655228852155959 ) ) ;
#21971=CARTESIAN_POINT ( 'NONE',  ( 0.4055118110236220486, 0.000000000000000000, 0.3543307086614173040 ) ) ;
#21977=EDGE_CURVE ( 'NONE', #7423, #17871, #14367, .T. ) ;
#21983=EDGE_CURVE ( 'NONE', #290, #2628, #18350, .T. ) ;
#22006=AXIS2_PLACEMENT_3D ( 'NONE', #15623, #24488, #24087 ) ;
#22010=ADVANCED_FACE ( 'NONE', ( #23108 ), #18841, .F. ) ;
#22011=DIRECTION ( 'NONE',  ( 0.000000000000000000, 1.000000000000000000, 0.000000000000000000 ) ) ;
#22013=EDGE_CURVE ( 'NONE', #3515, #22576, #3454, .T. ) ;
#22016=CARTESIAN_POINT ( 'NONE',  ( -0.3998447049182496382, 0.4754871227240771714, 0.09685039370078740717 ) ) ;
#22017=DIRECTION ( 'NONE',  ( 0.000000000000000000, 0.000000000000000000, 1.000000000000000000 ) ) ;
#22022=ORIENTED_EDGE ( 'NONE', *, *, #5186, .T. ) ;
#22035=CARTESIAN_POINT ( 'NONE',  ( 0.000000000000000000, 0.000000000000000000, 0.3059055118110236560 ) ) ;
#22040=CARTESIAN_POINT ( 'NONE',  ( -0.4246272423007197983, 0.5071139714526793352, 0.1926811207703575390 ) ) ;
#22049=MANIFOLD_SOLID_BREP ( 'Deep Groove Ball Bearing 20x37x9', #12801 ) ;
#22054=CIRCLE ( 'NONE', #3083, 0.5007874015748031704 ) ;
#22079=ORIENTED_EDGE ( 'NONE', *, *, #26746, .F. ) ;
#22081=DIRECTION ( 'NONE',  ( 0.000000000000000000, -1.000000000000000000, 0.000000000000000000 ) ) ;
#22085=CARTESIAN_POINT ( 'NONE',  ( -0.1579154690107267833, -0.4355388305873471588, 0.2048502515406250557 ) ) ;
#22089=CIRCLE ( 'NONE', #20751, 0.7283464566929134243 ) ;
#22099=SPHERICAL_SURFACE ( 'NONE', #2304, 0.1003956692913385851 ) ;
#22100=CARTESIAN_POINT ( 'NONE',  ( 0.0005710523241079800989, 0.4632828964885310485, 0.1494804572073301641 ) ) ;
#22107=CARTESIAN_POINT ( 'NONE',  ( 0.3131893444311545371, 0.3723335979429350795, 0.1075369453526922314 ) ) ;
#22108=CARTESIAN_POINT ( 'NONE',  ( 0.6512499169099681406, 0.1155267097730202641, 0.1616495878900666150 ) ) ;
#22113=AXIS2_PLACEMENT_3D ( 'NONE', #26529, #3075, #9294 ) ;
#22122=CARTESIAN_POINT ( 'NONE',  ( 0.0004405150045870399964, 0.6212597256746514862, 0.09684874924366457249 ) ) ;
#22131=B_SPLINE_CURVE_WITH_KNOTS ( 'NONE', 3,
 ( #19731, #8579, #15506, #23708, #14960, #2620, #11242, #6464, #4208, #15097 ),
 .UNSPECIFIED., .F., .F.,
 ( 4, 2, 2, 2, 4 ),
 ( 0.000000000000000000, 0.2500000000000000000, 0.5000000000000000000, 0.7500000000000000000, 1.000000000000000000 ),
 .UNSPECIFIED. ) ;
#22147=CARTESIAN_POINT ( 'NONE',  ( 0.000000000000000000, 0.000000000000000000, 0.1771653543307086520 ) ) ;
#22156=AXIS2_PLACEMENT_3D ( 'NONE', #23705, #26217, #15094 ) ;
#22169=CARTESIAN_POINT ( 'NONE',  ( 0.000000000000000000, 0.000000000000000000, 0.01181102362204724393 ) ) ;
#22173=CARTESIAN_POINT ( 'NONE',  ( -0.4339912984563299436, -0.2498791196563492356, 0.2574803149606298969 ) ) ;
#22193=EDGE_CURVE ( 'NONE', #4851, #3160, #2193, .T. ) ;
#22194=CARTESIAN_POINT ( 'NONE',  ( 0.1570092758121679200, -0.4330450457732857861, 0.1771653543307087630 ) ) ;
#22197=EDGE_CURVE ( 'NONE', #2702, #14152, #9942, .T. ) ;
#22200=B_SPLINE_CURVE_WITH_KNOTS ( 'NONE', 3,
 ( #19606, #6333, #25544, #12678, #4348, #21165 ),
 .UNSPECIFIED., .F., .F.,
 ( 4, 2, 4 ),
 ( 0.000000000000000000, 0.2500000000000000000, 0.5000000000000000000 ),
 .UNSPECIFIED. ) ;
#22201=SPHERICAL_SURFACE ( 'NONE', #26111, 0.1003956692913385851 ) ;
#22211=DIRECTION ( 'NONE',  ( 1.000000000000000000, 0.000000000000000000, 0.000000000000000000 ) ) ;
#22212=DIRECTION ( 'NONE',  ( 0.000000000000000000, 0.000000000000000000, 1.000000000000000000 ) ) ;
#22213=DIRECTION ( 'NONE',  ( 0.000000000000000000, 0.000000000000000000, 1.000000000000000000 ) ) ;
#22235=DIRECTION ( 'NONE',  ( 1.000000000000000000, 0.000000000000000000, 0.000000000000000000 ) ) ;
#22242=ORIENTED_EDGE ( 'NONE', *, *, #25261, .T. ) ;
#22254=CIRCLE ( 'NONE', #4231, 0.1003956692913385573 ) ;
#22267=CARTESIAN_POINT ( 'NONE',  ( 0.000000000000000000, 0.000000000000000000, 0.3059055118110236560 ) ) ;
#22290=CARTESIAN_POINT ( 'NONE',  ( 0.2161007281672546465, -0.5956855348316323351, 0.1061598535656166492 ) ) ;
#22297=EDGE_CURVE ( 'NONE', #17285, #11455, #17643, .T. ) ;
#22299=AXIS2_PLACEMENT_3D ( 'NONE', #17081, #16946, #23167 ) ;
#22305=EDGE_CURVE ( 'NONE', #24688, #20284, #15330, .T. ) ;
#22308=CARTESIAN_POINT ( 'NONE',  ( -0.0005855335178309040850, 0.4865383137632814381, 0.2467937632985283125 ) ) ;
#22318=AXIS2_PLACEMENT_3D ( 'NONE', #10905, #26693, #18346 ) ;
#22324=CARTESIAN_POINT ( 'NONE',  ( 0.000000000000000000, 0.000000000000000000, 0.01181102362204724393 ) ) ;
#22327=B_SPLINE_CURVE_WITH_KNOTS ( 'NONE', 3,
 ( #12452, #23352, #3976, #1852, #27714, #7935 ),
 .UNSPECIFIED., .F., .F.,
 ( 4, 2, 4 ),
 ( 0.5000000000000000000, 0.7500000000000000000, 1.000000000000000000 ),
 .UNSPECIFIED. ) ;
#22331=DIRECTION ( 'NONE',  ( 0.000000000000000000, 1.000000000000000000, 0.000000000000000000 ) ) ;
#22339=AXIS2_PLACEMENT_3D ( 'NONE', #3836, #21064, #27287 ) ;
#22344=ORIENTED_EDGE ( 'NONE', *, *, #14142, .F. ) ;
#22352=CARTESIAN_POINT ( 'NONE',  ( 0.000000000000000000, 0.000000000000000000, 0.09685039370078740717 ) ) ;
#22353=DIRECTION ( 'NONE',  ( -0.7660444431189780135, -0.6427876096865392519, 0.000000000000000000 ) ) ;
#22363=CARTESIAN_POINT ( 'NONE',  ( -0.5699748819085075358, -0.3282885190152641242, 0.1461456498326136888 ) ) ;
#22364=CIRCLE ( 'NONE', #25548, 0.6212598425196850238 ) ;
#22390=ORIENTED_EDGE ( 'NONE', *, *, #6615, .T. ) ;
#22391=EDGE_LOOP ( 'NONE', ( #12505, #21649, #2509, #11088, #1252, #6832, #14682, #21077, #18610, #13020, #23710, #5872, #11872, #19880 ) ) ;
#22404=ORIENTED_EDGE ( 'NONE', *, *, #1101, .T. ) ;
#22427=DIRECTION ( 'NONE',  ( 0.000000000000000000, 0.000000000000000000, 1.000000000000000000 ) ) ;
#22432=CARTESIAN_POINT ( 'NONE',  ( 0.3986320731132086959, -0.2308081338369904478, 0.1771653543307089018 ) ) ;
#22439=ORIENTED_EDGE ( 'NONE', *, *, #22642, .F. ) ;
#22455=CARTESIAN_POINT ( 'NONE',  ( -0.3988311005573527690, 0.4763376377694653607, 0.2574803149606298969 ) ) ;
#22461=CARTESIAN_POINT ( 'NONE',  ( 0.4339912984563291110, -0.2498791196563492356, 0.09685039370078740717 ) ) ;
#22475=ORIENTED_EDGE ( 'NONE', *, *, #11319, .F. ) ;
#22479=EDGE_CURVE ( 'NONE', #17871, #21791, #2479, .T. ) ;
#22495=DIRECTION ( 'NONE',  ( 0.000000000000000000, 1.000000000000000000, 0.000000000000000000 ) ) ;
#22530=ORIENTED_EDGE ( 'NONE', *, *, #18612, .T. ) ;
#22539=ORIENTED_EDGE ( 'NONE', *, *, #3464, .F. ) ;
#22540=CIRCLE ( 'NONE', #10359, 0.1003937007874015908 ) ;
#22549=ORIENTED_EDGE ( 'NONE', *, *, #3742, .T. ) ;
#22559=AXIS2_PLACEMENT_3D ( 'NONE', #3896, #23549, #12516 ) ;
#22563=CARTESIAN_POINT ( 'NONE',  ( 0.6119360453657125554, 0.1072290460171897442, 0.09685039370078740717 ) ) ;
#22567=CARTESIAN_POINT ( 'NONE',  ( -0.4535326485287285991, 0.08054850140359781641, 0.1639447408838820286 ) ) ;
#22576=VERTEX_POINT ( 'NONE', #4916 ) ;
#22591=CARTESIAN_POINT ( 'NONE',  ( -0.1634143070178008805, -0.4472844159266942121, 0.2330651858521301523 ) ) ;
#22592=CARTESIAN_POINT ( 'NONE',  ( 0.5381367953593070297, -0.3104394140547551140, 0.09684793308443542803 ) ) ;
#22608=CIRCLE ( 'NONE', #27134, 0.6212598425196850238 ) ;
#22610=ORIENTED_EDGE ( 'NONE', *, *, #26022, .F. ) ;
#22624=CIRCLE ( 'NONE', #24874, 0.4606299212598425341 ) ;
#22626=DIRECTION ( 'NONE',  ( 1.000000000000000000, 0.000000000000000000, 0.000000000000000000 ) ) ;
#22636=CARTESIAN_POINT ( 'NONE',  ( 0.000000000000000000, 0.000000000000000000, 0.01181102362204724393 ) ) ;
#22638=FACE_BOUND ( 'NONE', #1482, .T. ) ;
#22642=EDGE_CURVE ( 'NONE', #9472, #24177, #7905, .T. ) ;
#22643=CARTESIAN_POINT ( 'NONE',  ( 0.3217486617182078734, 0.3837523410419874659, 0.2574827755769819038 ) ) ;
#22647=DIRECTION ( 'NONE',  ( 0.8660254037844385966, -0.5000000000000003331, 0.000000000000000000 ) ) ;
#22648=CARTESIAN_POINT ( 'NONE',  ( -0.6119360453657125554, 0.1072290460171901605, 0.09685039370078740717 ) ) ;
#22656=FACE_OUTER_BOUND ( 'NONE', #2331, .T. ) ;
#22691=VERTEX_POINT ( 'NONE', #11984 ) ;
#22701=CARTESIAN_POINT ( 'NONE',  ( -0.4055118110236220486, 4.966087413865251393E-17, 0.01181102362204724393 ) ) ;
#22703=CARTESIAN_POINT ( 'NONE',  ( 0.5379168165870354956, -0.3108204284649153659, 0.2574827755769819038 ) ) ;
#22726=CARTESIAN_POINT ( 'NONE',  ( 0.4930758245789425009, 0.08754571829529310401, 0.2574803149606298969 ) ) ;
#22735=CIRCLE ( 'NONE', #25446, 0.5007874015748031704 ) ;
#22738=FACE_OUTER_BOUND ( 'NONE', #23269, .T. ) ;
#22765=CARTESIAN_POINT ( 'NONE',  ( -0.4932136069632142017, 0.08676634416062008193, 0.2574827755769819038 ) ) ;
#22774=LINE ( 'NONE', #9776, #26344 ) ;
#22791=ORIENTED_EDGE ( 'NONE', *, *, #1132, .T. ) ;
#22794=CARTESIAN_POINT ( 'NONE',  ( 0.5579526598169843865, -0.3213561723284312777, 0.2359405056216625773 ) ) ;
#22804=EDGE_CURVE ( 'NONE', #18356, #6451, #3167, .T. ) ;
#22815=EDGE_CURVE ( 'NONE', #8924, #12716, #18996, .T. ) ;
#22825=CARTESIAN_POINT ( 'NONE',  ( 0.000000000000000000, 0.000000000000000000, 0.09685039370078740717 ) ) ;
#22838=CARTESIAN_POINT ( 'NONE',  ( -0.2982299571017541506, 0.3545282230882351171, 0.1494804572094046713 ) ) ;
#22851=ORIENTED_EDGE ( 'NONE', *, *, #26400, .F. ) ;
#22867=ORIENTED_EDGE ( 'NONE', *, *, #6112, .T. ) ;
#22901=VERTEX_POINT ( 'NONE', #15234 ) ;
#22907=ORIENTED_EDGE ( 'NONE', *, *, #16318, .T. ) ;
#22917=VERTEX_POINT ( 'NONE', #17474 ) ;
#22923=CARTESIAN_POINT ( 'NONE',  ( -0.0006615832606325197825, 0.6212594902576319411, 0.09685039370078740717 ) ) ;
#22927=CARTESIAN_POINT ( 'NONE',  ( -0.6119360453657027854, 0.1072290460172413279, 0.2574803149606298969 ) ) ;
#22933=ORIENTED_EDGE ( 'NONE', *, *, #23684, .T. ) ;
#22940=ORIENTED_EDGE ( 'NONE', *, *, #27121, .T. ) ;
#22945=FACE_OUTER_BOUND ( 'NONE', #3690, .T. ) ;
#22947=CARTESIAN_POINT ( 'NONE',  ( 0.000000000000000000, 0.5610236220472440971, 0.1771653543307086520 ) ) ;
#22998=CARTESIAN_POINT ( 'NONE',  ( -0.5383572925355968319, -0.3100567972183898013, 0.09685039370078740717 ) ) ;
#22999=DIRECTION ( 'NONE',  ( 0.000000000000000000, 0.000000000000000000, -1.000000000000000000 ) ) ;
#23000=AXIS2_PLACEMENT_3D ( 'NONE', #19411, #13175, #13051 ) ;
#23010=CARTESIAN_POINT ( 'NONE',  ( 0.1580799066051618851, -0.4326553680327471785, 0.1771653543307085410 ) ) ;
#23013=CARTESIAN_POINT ( 'NONE',  ( 0.4535326485287340947, 0.08054850140356764610, 0.1903859678014195589 ) ) ;
#23014=ADVANCED_FACE ( 'NONE', ( #9396 ), #11530, .T. ) ;
#23038=TOROIDAL_SURFACE ( 'NONE', #14477, 0.5610236220472440971, 0.1003937007874015908 ) ;
#23041=VERTEX_POINT ( 'NONE', #5603 ) ;
#23042=EDGE_CURVE ( 'NONE', #3818, #2008, #2472, .T. ) ;
#23046=CARTESIAN_POINT ( 'NONE',  ( 0.000000000000000000, 0.000000000000000000, 0.1771653543307086520 ) ) ;
#23047=DIRECTION ( 'NONE',  ( 0.000000000000000000, 0.000000000000000000, 1.000000000000000000 ) ) ;
#23049=VERTEX_POINT ( 'NONE', #24654 ) ;
#23062=CARTESIAN_POINT ( 'NONE',  ( -0.6478824768862475603, 0.1135474080046062623, 0.1461456498260605696 ) ) ;
#23074=ORIENTED_EDGE ( 'NONE', *, *, #23876, .T. ) ;
#23101=VERTEX_POINT ( 'NONE', #21133 ) ;
#23108=FACE_OUTER_BOUND ( 'NONE', #9775, .T. ) ;
#23125=DIRECTION ( 'NONE',  ( -0.9396926207859083169, -0.3420201433256692125, 0.000000000000000000 ) ) ;
#23127=AXIS2_PLACEMENT_3D ( 'NONE', #19436, #1783, #131 ) ;
#23133=CARTESIAN_POINT ( 'NONE',  ( 0.0006681923949024700608, 0.6336721034114674023, 0.2481708550952533565 ) ) ;
#23144=CARTESIAN_POINT ( 'NONE',  ( -0.2268599607415002495, -0.6212949646971562823, 0.1926811207740130039 ) ) ;
#23166=CARTESIAN_POINT ( 'NONE',  ( 0.5379168165870276130, -0.3108204284649302984, 0.09684793308443542803 ) ) ;
#23167=DIRECTION ( 'NONE',  ( 0.000000000000000000, 0.000000000000000000, -1.000000000000000000 ) ) ;
#23171=CARTESIAN_POINT ( 'NONE',  ( -0.3222028160008074682, 0.3833711078595924970, 0.2574819596263889787 ) ) ;
#23182=EDGE_CURVE ( 'NONE', #24915, #8070, #15292, .T. ) ;
#23207=CARTESIAN_POINT ( 'NONE',  ( 0.0005939837304750000086, 0.5007870493127504208, 0.2574803149606298969 ) ) ;
#23225=ORIENTED_EDGE ( 'NONE', *, *, #4810, .F. ) ;
#23232=DIRECTION ( 'NONE',  ( 0.000000000000000000, -1.000000000000000000, 0.000000000000000000 ) ) ;
#23236=EDGE_CURVE ( 'NONE', #15131, #12919, #6387, .T. ) ;
#23240=FACE_OUTER_BOUND ( 'NONE', #11247, .T. ) ;
#23249=AXIS2_PLACEMENT_3D ( 'NONE', #26338, #639, #23823 ) ;
#23268=SPHERICAL_SURFACE ( 'NONE', #22559, 0.1003956692913385851 ) ;
#23269=EDGE_LOOP ( 'NONE', ( #4610, #17340, #2215, #14699, #10174, #27172, #3533, #21565, #9322, #22851, #318, #21853, #14483, #27390 ) ) ;
#23296=ORIENTED_EDGE ( 'NONE', *, *, #14142, .T. ) ;
#23298=ORIENTED_EDGE ( 'NONE', *, *, #13512, .F. ) ;
#23302=EDGE_CURVE ( 'NONE', #24919, #1804, #17000, .T. ) ;
#23314=ORIENTED_EDGE ( 'NONE', *, *, #2233, .F. ) ;
#23318=DIRECTION ( 'NONE',  ( 0.000000000000000000, 1.000000000000000000, 0.000000000000000000 ) ) ;
#23327=CIRCLE ( 'NONE', #12469, 0.1003956692913385990 ) ;
#23333=CARTESIAN_POINT ( 'NONE',  ( 0.4606299212598425341, 0.000000000000000000, 0.1771653543307086520 ) ) ;
#23336=ORIENTED_EDGE ( 'NONE', *, *, #8618, .T. ) ;
#23340=CARTESIAN_POINT ( 'NONE',  ( 0.1714649452450068834, -0.4705186852026070898, 0.09684793308443542803 ) ) ;
#23346=ORIENTED_EDGE ( 'NONE', *, *, #21415, .F. ) ;
#23352=CARTESIAN_POINT ( 'NONE',  ( 0.4537304931026565069, 0.07942646906837147469, 0.1903859678062056193 ) ) ;
#23353=DIRECTION ( 'NONE',  ( 0.000000000000000000, 1.000000000000000000, 0.000000000000000000 ) ) ;
#23381=DIRECTION ( 'NONE',  ( 0.000000000000000000, 0.000000000000000000, 1.000000000000000000 ) ) ;
#23385=CARTESIAN_POINT ( 'NONE',  ( -0.2128972891168988413, -0.5836425148029299459, 0.2574819594177527593 ) ) ;
#23397=EDGE_CURVE ( 'NONE', #27022, #3924, #18160, .T. ) ;
#23400=TOROIDAL_SURFACE ( 'NONE', #11195, 0.4055118110236220486, 0.01181102362204724393 ) ;
#23401=CARTESIAN_POINT ( 'NONE',  ( 0.4932821129636645874, 0.08637579872942321990, 0.2574803149606298969 ) ) ;
#23403=CARTESIAN_POINT ( 'NONE',  ( 0.2208527687061731248, -0.6048181665932198525, 0.1183902030356892010 ) ) ;
#23453=ORIENTED_EDGE ( 'NONE', *, *, #12450, .T. ) ;
#23463=CIRCLE ( 'NONE', #14895, 0.6212598425196850238 ) ;
#23464=CARTESIAN_POINT ( 'NONE',  ( 0.000000000000000000, 0.5007874015748031704, 0.3543307086614173040 ) ) ;
#23483=ORIENTED_EDGE ( 'NONE', *, *, #5518, .F. ) ;
#23493=ORIENTED_EDGE ( 'NONE', *, *, #26022, .T. ) ;
#23494=DIRECTION ( 'NONE',  ( 1.000000000000000000, 0.000000000000000000, 0.000000000000000000 ) ) ;
#23515=CYLINDRICAL_SURFACE ( 'NONE', #15761, 0.3937007874015748254 ) ;
#23518=CARTESIAN_POINT ( 'NONE',  ( 0.4246272423004305296, 0.5071139714523401620, 0.1616495878881752113 ) ) ;
#23544=EDGE_CURVE ( 'NONE', #6246, #2628, #6540, .T. ) ;
#23549=DIRECTION ( 'NONE',  ( 0.000000000000000000, 1.000000000000000000, 0.000000000000000000 ) ) ;
#23551=CARTESIAN_POINT ( 'NONE',  ( 0.000000000000000000, 0.000000000000000000, 0.2574803149606298969 ) ) ;
#23556=CARTESIAN_POINT ( 'NONE',  ( -0.3606190329934327310, 0.4297690281277732338, 0.1771653543307086520 ) ) ;
#23557=DIRECTION ( 'NONE',  ( 0.000000000000000000, 1.000000000000000000, 0.000000000000000000 ) ) ;
#23577=CARTESIAN_POINT ( 'NONE',  ( -0.3998447049182496382, 0.4754871227240771714, 0.09685039370078740717 ) ) ;
#23579=FACE_OUTER_BOUND ( 'NONE', #6640, .T. ) ;
#23606=CARTESIAN_POINT ( 'NONE',  ( -0.0001974756197917525776, 0.5007874015748032814, 0.2574827755769819038 ) ) ;
#23609=CARTESIAN_POINT ( 'NONE',  ( 0.1580799066051618851, -0.4326553680327471785, 0.1771653543307085410 ) ) ;
#23619=EDGE_CURVE ( 'NONE', #798, #9216, #6935, .T. ) ;
#23620=CARTESIAN_POINT ( 'NONE',  ( -0.5525004126151165096, 0.09742072959660473541, 0.2775610236220472093 ) ) ;
#23629=CARTESIAN_POINT ( 'NONE',  ( 0.6342142812959871145, 0.1111449751014438880, 0.2359405056220046093 ) ) ;
#23651=ADVANCED_FACE ( 'NONE', ( #24987 ), #16854, .T. ) ;
#23654=CARTESIAN_POINT ( 'NONE',  ( -0.3988311005573527690, 0.4763376377694653607, 0.2574803149606298969 ) ) ;
#23657=DIRECTION ( 'NONE',  ( 0.000000000000000000, -1.000000000000000000, 0.000000000000000000 ) ) ;
#23658=VECTOR ( 'NONE', #22213, 39.37007874015748143 ) ;
#23677=CARTESIAN_POINT ( 'NONE',  ( 0.2256062985789750452, -0.6178563876572671365, 0.2081850588211440756 ) ) ;
#23684=EDGE_CURVE ( 'NONE', #21791, #16455, #10219, .T. ) ;
#23690=EDGE_CURVE ( 'NONE', #11735, #17779, #19576, .T. ) ;
#23696=CARTESIAN_POINT ( 'NONE',  ( -0.6117448998508603353, 0.1083144418130620040, 0.2574819594177531479 ) ) ;
#23700=ORIENTED_EDGE ( 'NONE', *, *, #6090, .F. ) ;
#23702=CARTESIAN_POINT ( 'NONE',  ( 0.4537304931026562849, 0.07942646906837143306, 0.1771653543307087630 ) ) ;
#23705=CARTESIAN_POINT ( 'NONE',  ( 0.000000000000000000, 0.000000000000000000, 0.09685039370078740717 ) ) ;
#23708=CARTESIAN_POINT ( 'NONE',  ( -0.6476458834297724731, 0.1148891961921066213, 0.2081850588258900292 ) ) ;
#23710=ORIENTED_EDGE ( 'NONE', *, *, #233, .T. ) ;
#23720=CARTESIAN_POINT ( 'NONE',  ( 0.6117833106355984318, 0.1080972763116263835, 0.09684793308443542803 ) ) ;
#23768=DIRECTION ( 'NONE',  ( 0.000000000000000000, 1.000000000000000000, 0.000000000000000000 ) ) ;
#23775=AXIS2_PLACEMENT_3D ( 'NONE', #14328, #25862, #3713 ) ;
#23780=CARTESIAN_POINT ( 'NONE',  ( -0.3986320731132245165, -0.2308081338369633029, 0.1639447408623057878 ) ) ;
#23787=CARTESIAN_POINT ( 'NONE',  ( 0.4068047116061080937, 0.4858504993705154984, 0.2481708550949471570 ) ) ;
#23793=CARTESIAN_POINT ( 'NONE',  ( 0.000000000000000000, 0.000000000000000000, 0.2574803149606298969 ) ) ;
#23803=EDGE_LOOP ( 'NONE', ( #4282, #16678, #18782, #19992, #13296, #19117 ) ) ;
#23823=DIRECTION ( 'NONE',  ( 0.000000000000000000, 1.000000000000000000, 0.000000000000000000 ) ) ;
#23829=DIRECTION ( 'NONE',  ( -0.6427876096865390299, 0.7660444431189783465, 0.000000000000000000 ) ) ;
#23837=CARTESIAN_POINT ( 'NONE',  ( 0.4537304931026565069, 0.07942646906837144694, 0.1639447408552120455 ) ) ;
#23842=EDGE_LOOP ( 'NONE', ( #20467, #18255 ) ) ;
#23847=ORIENTED_EDGE ( 'NONE', *, *, #27294, .F. ) ;
#23868=ORIENTED_EDGE ( 'NONE', *, *, #6090, .T. ) ;
#23876=EDGE_CURVE ( 'NONE', #1165, #13130, #1964, .T. ) ;
#23878=ORIENTED_EDGE ( 'NONE', *, *, #23302, .T. ) ;
#23879=CIRCLE ( 'NONE', #1741, 0.1003956692913385990 ) ;
#23880=CARTESIAN_POINT ( 'NONE',  ( -0.2973550541826790461, 0.3552623538052492869, 0.2048502514528301177 ) ) ;
#23882=DIRECTION ( 'NONE',  ( 0.000000000000000000, 1.000000000000000000, 0.000000000000000000 ) ) ;
#23891=VERTEX_POINT ( 'NONE', #7301 ) ;
#23893=EDGE_CURVE ( 'NONE', #2008, #833, #16398, .T. ) ;
#23915=ORIENTED_EDGE ( 'NONE', *, *, #5854, .F. ) ;
#23933=DIRECTION ( 'NONE',  ( 0.000000000000000000, 0.000000000000000000, -1.000000000000000000 ) ) ;
#23941=DIRECTION ( 'NONE',  ( 0.000000000000000000, 1.000000000000000000, 0.000000000000000000 ) ) ;
#23949=CARTESIAN_POINT ( 'NONE',  ( -0.3992017438595020229, -0.2298214351608249550, 0.1639447408619164881 ) ) ;
#23958=ORIENTED_EDGE ( 'NONE', *, *, #14545, .T. ) ;
#23974=ORIENTED_EDGE ( 'NONE', *, *, #6150, .T. ) ;
#23979=ORIENTED_EDGE ( 'NONE', *, *, #17844, .F. ) ;
#23985=B_SPLINE_CURVE_WITH_KNOTS ( 'NONE', 3,
 ( #15005, #6513, #25865, #2397, #11159, #19777 ),
 .UNSPECIFIED., .F., .F.,
 ( 4, 2, 4 ),
 ( 0.000000000000000000, 0.2500000000000000000, 0.5000000000000000000 ),
 .UNSPECIFIED. ) ;
#23992=EDGE_CURVE ( 'NONE', #20032, #20701, #5592, .T. ) ;
#24005=DIRECTION ( 'NONE',  ( 0.000000000000000000, 0.000000000000000000, -1.000000000000000000 ) ) ;
#24010=DIRECTION ( 'NONE',  ( 0.000000000000000000, 0.000000000000000000, 1.000000000000000000 ) ) ;
#24020=CIRCLE ( 'NONE', #19054, 0.01181102362204724046 ) ;
#24021=CARTESIAN_POINT ( 'NONE',  ( 0.1707210962531913734, -0.4707890492249701131, 0.09685039370078740717 ) ) ;
#24026=CARTESIAN_POINT ( 'NONE',  ( 0.000000000000000000, 0.000000000000000000, 0.1771653543307086520 ) ) ;
#24051=CARTESIAN_POINT ( 'NONE',  ( 0.1716509673353401599, -0.4704508543867079173, 0.09684874903502814492 ) ) ;
#24073=DIRECTION ( 'NONE',  ( 0.000000000000000000, 0.000000000000000000, 1.000000000000000000 ) ) ;
#24087=DIRECTION ( 'NONE',  ( 0.000000000000000000, 1.000000000000000000, 0.000000000000000000 ) ) ;
#24090=AXIS2_PLACEMENT_3D ( 'NONE', #14609, #1721, #12463 ) ;
#24111=AXIS2_PLACEMENT_3D ( 'NONE', #2775, #22017, #15930 ) ;
#24114=EDGE_LOOP ( 'NONE', ( #14967, #407, #21651, #11522, #12563, #25829 ) ) ;
#24128=CARTESIAN_POINT ( 'NONE',  ( 0.3214446924536846772, 0.3840069416942866742, 0.2574803149606298969 ) ) ;
#24130=CARTESIAN_POINT ( 'NONE',  ( -0.4333973147258542991, -0.2509079296564011852, 0.2574803149606298969 ) ) ;
#24144=ORIENTED_EDGE ( 'NONE', *, *, #6459, .T. ) ;
#24145=CARTESIAN_POINT ( 'NONE',  ( 0.000000000000000000, 0.000000000000000000, 0.3543307086614173040 ) ) ;
#24148=DIRECTION ( 'NONE',  ( 0.000000000000000000, 0.000000000000000000, 1.000000000000000000 ) ) ;
#24168=CARTESIAN_POINT ( 'NONE',  ( 0.3992017438595159562, -0.2298214351608004746, 0.1771653543307084855 ) ) ;
#24169=CARTESIAN_POINT ( 'NONE',  ( -0.1918813796216842782, -0.5271897577243779276, 0.1771653543307086520 ) ) ;
#24177=VERTEX_POINT ( 'NONE', #18624 ) ;
#24188=CARTESIAN_POINT ( 'NONE',  ( -0.6117833106355984318, 0.1080972763116267721, 0.09684793308443542803 ) ) ;
#24210=DIRECTION ( 'NONE',  ( 0.000000000000000000, 0.000000000000000000, 1.000000000000000000 ) ) ;
#24216=FACE_OUTER_BOUND ( 'NONE', #4481, .T. ) ;
#24219=AXIS2_PLACEMENT_3D ( 'NONE', #3737, #16598, #1483 ) ;
#24230=VERTEX_POINT ( 'NONE', #25754 ) ;
#24248=ORIENTED_EDGE ( 'NONE', *, *, #4448, .T. ) ;
#24249=ORIENTED_EDGE ( 'NONE', *, *, #11319, .T. ) ;
#24262=CARTESIAN_POINT ( 'NONE',  ( -0.4121125639576288524, -0.2386018002113109993, 0.2330651857992618037 ) ) ;
#24283=EDGE_LOOP ( 'NONE', ( #13919, #2353, #1704, #1896, #29, #16178 ) ) ;
#24286=CARTESIAN_POINT ( 'NONE',  ( -0.1580799066051627177, -0.4326553680327468454, 0.1771653543307088186 ) ) ;
#24301=ORIENTED_EDGE ( 'NONE', *, *, #19828, .F. ) ;
#24305=B_SPLINE_CURVE_WITH_KNOTS ( 'NONE', 3,
 ( #17140, #14907, #2292, #10631, #23518, #21660, #4148, #12757, #23787, #4558 ),
 .UNSPECIFIED., .F., .F.,
 ( 4, 2, 2, 2, 4 ),
 ( 0.000000000000000000, 0.2500000000000000000, 0.5000000000000000000, 0.7500000000000000000, 1.000000000000000000 ),
 .UNSPECIFIED. ) ;
#24338=CARTESIAN_POINT ( 'NONE',  ( -0.0006832381873107856631, 0.6614169699452854267, 0.1616495878891046900 ) ) ;
#24342=AXIS2_PLACEMENT_3D ( 'NONE', #17647, #24010, #6240 ) ;
#24345=ORIENTED_EDGE ( 'NONE', *, *, #19828, .T. ) ;
#24349=DIRECTION ( 'NONE',  ( -0.3420201433256691570, -0.9396926207859082059, 0.000000000000000000 ) ) ;
#24354=CIRCLE ( 'NONE', #3150, 0.6212598425196850238 ) ;
#24358=CARTESIAN_POINT ( 'NONE',  ( -0.4339912984563299436, -0.2498791196563492356, 0.09685039370078740717 ) ) ;
#24365=AXIS2_PLACEMENT_3D ( 'NONE', #14079, #8149, #5896 ) ;
#24376=CARTESIAN_POINT ( 'NONE',  ( 0.0002199787722797491975, 0.6212598425196850238, 0.09684793308443542803 ) ) ;
#24387=DIRECTION ( 'NONE',  ( 0.000000000000000000, 0.000000000000000000, 1.000000000000000000 ) ) ;
#24394=CARTESIAN_POINT ( 'NONE',  ( 0.6342142812972784149, 0.1111449751016729826, 0.1183902030411032036 ) ) ;
#24408=AXIS2_PLACEMENT_3D ( 'NONE', #22169, #5064, #26528 ) ;
#24435=AXIS2_PLACEMENT_3D ( 'NONE', #26437, #21794, #19399 ) ;
#24436=CARTESIAN_POINT ( 'NONE',  ( -0.7165354330708662012, 8.775028245858987528E-17, 0.3425196850393700809 ) ) ;
#24454=CARTESIAN_POINT ( 'NONE',  ( 0.6117062799105531523, 0.1085321106658064944, 0.2574803149606298969 ) ) ;
#24456=CARTESIAN_POINT ( 'NONE',  ( 0.000000000000000000, 0.5007874015748031704, 0.04842519685039370358 ) ) ;
#24459=CARTESIAN_POINT ( 'NONE',  ( 0.4858607088160724063, -0.2805118110236220486, 0.1771653543307086520 ) ) ;
#24466=B_SPLINE_CURVE_WITH_KNOTS ( 'NONE', 3,
 ( #23010, #18456, #1116, #12401, #12255, #11981 ),
 .UNSPECIFIED., .F., .F.,
 ( 4, 2, 4 ),
 ( 0.5000000000000000000, 0.7500000000000000000, 1.000000000000000000 ),
 .UNSPECIFIED. ) ;
#24488=DIRECTION ( 'NONE',  ( 0.000000000000000000, 0.000000000000000000, 1.000000000000000000 ) ) ;
#24500=ADVANCED_FACE ( 'NONE', ( #27598 ), #2454, .T. ) ;
#24505=ORIENTED_EDGE ( 'NONE', *, *, #19686, .T. ) ;
#24519=CARTESIAN_POINT ( 'NONE',  ( -0.2965233727166468047, 0.3524965443697193335, 0.1771653543307085965 ) ) ;
#24579=AXIS2_PLACEMENT_3D ( 'NONE', #11514, #393, #17597 ) ;
#24598=DIRECTION ( 'NONE',  ( 0.000000000000000000, 0.000000000000000000, 1.000000000000000000 ) ) ;
#24604=DIRECTION ( 'NONE',  ( 0.7660444431189780135, 0.6427876096865392519, 0.000000000000000000 ) ) ;
#24610=DIRECTION ( 'NONE',  ( 0.000000000000000000, 0.000000000000000000, 1.000000000000000000 ) ) ;
#24618=DIRECTION ( 'NONE',  ( 0.000000000000000000, 0.000000000000000000, 1.000000000000000000 ) ) ;
#24620=DIRECTION ( 'NONE',  ( 0.000000000000000000, -1.000000000000000000, 0.000000000000000000 ) ) ;
#24626=TOROIDAL_SURFACE ( 'NONE', #21489, 0.5610236220472440971, 0.1003937007874015908 ) ;
#24627=CARTESIAN_POINT ( 'NONE',  ( 0.0005939837304750000086, 0.5007870493127504208, 0.09685039370078740717 ) ) ;
#24649=CIRCLE ( 'NONE', #3453, 0.4055118110236220486 ) ;
#24654=CARTESIAN_POINT ( 'NONE',  ( 0.0005939837304750000086, 0.5007870493127504208, 0.2574803149606298969 ) ) ;
#24664=CARTESIAN_POINT ( 'NONE',  ( 0.6514872030416209991, 0.1141809932448827059, 0.1926811207754475230 ) ) ;
#24679=VERTEX_POINT ( 'NONE', #27401 ) ;
#24688=VERTEX_POINT ( 'NONE', #1395 ) ;
#24713=AXIS2_PLACEMENT_3D ( 'NONE', #6954, #17801, #22331 ) ;
#24718=VERTEX_POINT ( 'NONE', #25272 ) ;
#24720=CARTESIAN_POINT ( 'NONE',  ( -0.3220512119205936608, 0.3834984712787528061, 0.09684793308443542803 ) ) ;
#24728=CARTESIAN_POINT ( 'NONE',  ( -0.2118615749922956593, -0.5840192333899354438, 0.09685039370078740717 ) ) ;
#24729=CIRCLE ( 'NONE', #20218, 0.5007874015748031704 ) ;
#24742=DIRECTION ( 'NONE',  ( 1.000000000000000000, 0.000000000000000000, 0.000000000000000000 ) ) ;
#24754=EDGE_CURVE ( 'NONE', #21183, #19404, #19931, .T. ) ;
#24767=CARTESIAN_POINT ( 'NONE',  ( 0.000000000000000000, 0.000000000000000000, 0.3543307086614173040 ) ) ;
#24786=ORIENTED_EDGE ( 'NONE', *, *, #15046, .T. ) ;
#24787=AXIS2_PLACEMENT_3D ( 'NONE', #772, #1057, #24620 ) ;
#24794=EDGE_CURVE ( 'NONE', #16332, #8070, #12879, .T. ) ;
#24795=ORIENTED_EDGE ( 'NONE', *, *, #4503, .T. ) ;
#24802=DIRECTION ( 'NONE',  ( 0.000000000000000000, 1.000000000000000000, 0.000000000000000000 ) ) ;
#24812=B_SPLINE_CURVE_WITH_KNOTS ( 'NONE', 3,
 ( #5000, #26609, #15885, #24627 ),
 .UNSPECIFIED., .F., .F.,
 ( 4, 4 ),
 ( 0.3015484798814578316, 0.3030532441042709801 ),
 .UNSPECIFIED. ) ;
#24814=CARTESIAN_POINT ( 'NONE',  ( 0.5383572925355708527, -0.3100567972184350429, 0.2574803149606298969 ) ) ;
#24816=DIRECTION ( 'NONE',  ( 0.000000000000000000, 0.000000000000000000, 1.000000000000000000 ) ) ;
#24817=CARTESIAN_POINT ( 'NONE',  ( -0.5378064472801062923, -0.3110113600220464902, 0.09684874924366436433 ) ) ;
#24829=CARTESIAN_POINT ( 'NONE',  ( 0.2255758929760254272, -0.6217623271433985188, 0.1926811207689738403 ) ) ;
#24838=ORIENTED_EDGE ( 'NONE', *, *, #18061, .F. ) ;
#24840=EDGE_CURVE ( 'NONE', #4007, #17345, #25459, .T. ) ;
#24856=DIRECTION ( 'NONE',  ( 0.8660254037844387076, 0.4999999999999998890, -0.000000000000000000 ) ) ;
#24869=DIRECTION ( 'NONE',  ( 0.000000000000000000, 0.000000000000000000, 1.000000000000000000 ) ) ;
#24874=AXIS2_PLACEMENT_3D ( 'NONE', #1422, #14744, #12155 ) ;
#24876=DIRECTION ( 'NONE',  ( 0.000000000000000000, 0.000000000000000000, 1.000000000000000000 ) ) ;
#24881=CARTESIAN_POINT ( 'NONE',  ( -0.4930758245789425009, 0.08754571829529331217, 0.2574803149606298969 ) ) ;
#24898=FACE_OUTER_BOUND ( 'NONE', #7211, .T. ) ;
#24905=CARTESIAN_POINT ( 'NONE',  ( 0.5699748819085377338, -0.3282885190152939336, 0.1461456498327310671 ) ) ;
#24912=LINE ( 'NONE', #20399, #12098 ) ;
#24915=VERTEX_POINT ( 'NONE', #2640 ) ;
#24919=VERTEX_POINT ( 'NONE', #13109 ) ;
#24933=EDGE_LOOP ( 'NONE', ( #13430, #4494, #26526, #17444 ) ) ;
#24940=EDGE_LOOP ( 'NONE', ( #1022, #27456, #20518, #20289 ) ) ;
#24956=CARTESIAN_POINT ( 'NONE',  ( -0.5383572925356228112, -0.3100567972183445042, 0.2574803149606298969 ) ) ;
#24959=CARTESIAN_POINT ( 'NONE',  ( 0.000000000000000000, 0.5610236220472440971, -3.341531889763779686E-17 ) ) ;
#24961=AXIS2_PLACEMENT_3D ( 'NONE', #958, #9545, #11820 ) ;
#24982=DIRECTION ( 'NONE',  ( 0.000000000000000000, 0.000000000000000000, 1.000000000000000000 ) ) ;
#24984=DIRECTION ( 'NONE',  ( 0.000000000000000000, 0.000000000000000000, 1.000000000000000000 ) ) ;
#24987=FACE_OUTER_BOUND ( 'NONE', #21306, .T. ) ;
#24998=VERTEX_POINT ( 'NONE', #13945 ) ;
#25017=CARTESIAN_POINT ( 'NONE',  ( -0.6241612307011117355, 0.1093779649451541158, 0.2481708550935493307 ) ) ;
#25019=ORIENTED_EDGE ( 'NONE', *, *, #15940, .F. ) ;
#25038=SPHERICAL_SURFACE ( 'NONE', #21005, 0.1003956692913385851 ) ;
#25054=ORIENTED_EDGE ( 'NONE', *, *, #25456, .T. ) ;
#25056=CARTESIAN_POINT ( 'NONE',  ( -0.2131049448084480213, -0.5835666837866708700, 0.2574803149606298969 ) ) ;
#25060=ORIENTED_EDGE ( 'NONE', *, *, #8485, .T. ) ;
#25073=CARTESIAN_POINT ( 'NONE',  ( -0.2956505864974143805, 0.3532288989643738719, 0.1771653543307089018 ) ) ;
#25088=CIRCLE ( 'NONE', #2540, 0.01181102362204724046 ) ;
#25101=CARTESIAN_POINT ( 'NONE',  ( 0.3937007874015748254, 0.000000000000000000, 0.01181102362204724393 ) ) ;
#25105=ORIENTED_EDGE ( 'NONE', *, *, #22479, .T. ) ;
#25113=VERTEX_POINT ( 'NONE', #18297 ) ;
#25119=ORIENTED_EDGE ( 'NONE', *, *, #969, .T. ) ;
#25126=CARTESIAN_POINT ( 'NONE',  ( 0.000000000000000000, 0.000000000000000000, 0.2574803149606298969 ) ) ;
#25134=UNCERTAINTY_MEASURE_WITH_UNIT (LENGTH_MEASURE( 1.000000000000000082E-05 ), #14651, 'distance_accuracy_value', 'NONE') ;
#25147=ORIENTED_EDGE ( 'NONE', *, *, #21762, .T. ) ;
#25166=DIRECTION ( 'NONE',  ( 1.000000000000000000, 0.000000000000000000, 0.000000000000000000 ) ) ;
#25190=DIRECTION ( 'NONE',  ( 0.000000000000000000, -1.000000000000000000, 0.000000000000000000 ) ) ;
#25203=CIRCLE ( 'NONE', #13475, 0.5007874015748031704 ) ;
#25236=EDGE_CURVE ( 'NONE', #23049, #24998, #27710, .T. ) ;
#25239=CARTESIAN_POINT ( 'NONE',  ( 0.5378064472801236118, -0.3110113600220169028, 0.2574819594177531479 ) ) ;
#25248=CARTESIAN_POINT ( 'NONE',  ( -0.5525004126151165096, 0.09742072959660473541, 0.1771653543307086520 ) ) ;
#25250=CARTESIAN_POINT ( 'NONE',  ( -0.2173565190931825430, -0.5952284643153563648, 0.2481708550949385528 ) ) ;
#25253=ORIENTED_EDGE ( 'NONE', *, *, #11636, .T. ) ;
#25259=ORIENTED_EDGE ( 'NONE', *, *, #2902, .T. ) ;
#25261=EDGE_CURVE ( 'NONE', #5673, #4739, #1576, .T. ) ;
#25270=DIRECTION ( 'NONE',  ( 1.000000000000000000, 0.000000000000000000, 0.000000000000000000 ) ) ;
#25272=CARTESIAN_POINT ( 'NONE',  ( -2.184900367198595585E-17, 0.6212598425196850238, 0.2574827755769818483 ) ) ;
#25282=CARTESIAN_POINT ( 'NONE',  ( 0.2965233727166233235, 0.3524965443697389844, 0.1903859678001459665 ) ) ;
#25287=ORIENTED_EDGE ( 'NONE', *, *, #14509, .T. ) ;
#25292=CARTESIAN_POINT ( 'NONE',  ( -0.3214446924536846772, 0.3840069416942866742, 0.09685039370078740717 ) ) ;
#25300=CARTESIAN_POINT ( 'NONE',  ( -0.2118615749922468650, -0.5840192333899535404, 0.2574803149606298969 ) ) ;
#25301=CARTESIAN_POINT ( 'NONE',  ( 0.000000000000000000, 0.000000000000000000, 0.1771653543307086520 ) ) ;
#25303=CIRCLE ( 'NONE', #13120, 0.4055118110236220486 ) ;
#25328=ORIENTED_EDGE ( 'NONE', *, *, #11322, .F. ) ;
#25374=CARTESIAN_POINT ( 'NONE',  ( 0.000000000000000000, 0.000000000000000000, 0.3543307086614173040 ) ) ;
#25396=EDGE_CURVE ( 'NONE', #23101, #6477, #26370, .T. ) ;
#25397=CARTESIAN_POINT ( 'NONE',  ( -0.3998447049182095037, 0.4754871227241110332, 0.2574803149606298969 ) ) ;
#25411=CARTESIAN_POINT ( 'NONE',  ( -0.4930758245789425009, 0.08754571829529331217, 0.2574803149606298969 ) ) ;
#25423=EDGE_CURVE ( 'NONE', #12635, #13218, #11129, .T. ) ;
#25425=CARTESIAN_POINT ( 'NONE',  ( -6.132876883919029269E-17, -0.5007874015748031704, 0.3543307086614173040 ) ) ;
#25427=CARTESIAN_POINT ( 'NONE',  ( -0.0003954787107570180166, 0.5007872847596378518, 0.2574819596263889787 ) ) ;
#25446=AXIS2_PLACEMENT_3D ( 'NONE', #27021, #14307, #7666 ) ;
#25447=CARTESIAN_POINT ( 'NONE',  ( -0.1716509673353403542, -0.4704508543867079173, 0.2574819596263889787 ) ) ;
#25449=DIRECTION ( 'NONE',  ( 1.000000000000000000, 0.000000000000000000, 0.000000000000000000 ) ) ;
#25456=EDGE_CURVE ( 'NONE', #11052, #15868, #26994, .T. ) ;
#25459=CIRCLE ( 'NONE', #22299, 0.01181102362204724393 ) ;
#25468=ORIENTED_EDGE ( 'NONE', *, *, #26914, .F. ) ;
#25470=EDGE_CURVE ( 'NONE', #14064, #16082, #17539, .T. ) ;
#25471=CARTESIAN_POINT ( 'NONE',  ( -0.4009292313432017418, -0.2321359940680557676, 0.1494804571774004665 ) ) ;
#25476=VERTEX_POINT ( 'NONE', #12032 ) ;
#25482=CARTESIAN_POINT ( 'NONE',  ( 0.000000000000000000, 0.000000000000000000, 0.01181102362204724393 ) ) ;
#25495=TOROIDAL_SURFACE ( 'NONE', #6543, 0.5610236220472440971, 0.1003937007874015908 ) ;
#25499=AXIS2_PLACEMENT_3D ( 'NONE', #6376, #19367, #18683 ) ;
#25502=SURFACE_SIDE_STYLE ('',( #14353 ) ) ;
#25512=EDGE_LOOP ( 'NONE', ( #145, #13493, #12175, #5877 ) ) ;
#25530=DIRECTION ( 'NONE',  ( 0.000000000000000000, 0.000000000000000000, 1.000000000000000000 ) ) ;
#25531=DIRECTION ( 'NONE',  ( 0.000000000000000000, 0.000000000000000000, 1.000000000000000000 ) ) ;
#25538=ORIENTED_EDGE ( 'NONE', *, *, #4541, .T. ) ;
#25540=AXIS2_PLACEMENT_3D ( 'NONE', #6133, #2421, #8381 ) ;
#25544=CARTESIAN_POINT ( 'NONE',  ( -0.3065394984460679817, 0.3644188802930369842, 0.2330651857766198043 ) ) ;
#25548=AXIS2_PLACEMENT_3D ( 'NONE', #10760, #15438, #23768 ) ;
#25558=CARTESIAN_POINT ( 'NONE',  ( -0.3606190329934327310, 0.4297690281277732338, 0.1771653543307086520 ) ) ;
#25561=EDGE_CURVE ( 'NONE', #14369, #27683, #13327, .T. ) ;
#25587=LINE ( 'NONE', #6242, #8654 ) ;
#25588=CARTESIAN_POINT ( 'NONE',  ( -0.4537304931026616139, 0.07942646906834205378, 0.1771653543307086243 ) ) ;
#25599=( GEOMETRIC_REPRESENTATION_CONTEXT ( 3 ) GLOBAL_UNCERTAINTY_ASSIGNED_CONTEXT ( ( #3650 ) ) GLOBAL_UNIT_ASSIGNED_CONTEXT ( ( #13265, #17890, #15670 ) ) REPRESENTATION_CONTEXT ( 'NONE', 'WORKASPACE' ) ) ;
#25619=DIRECTION ( 'NONE',  ( 0.000000000000000000, 0.000000000000000000, 1.000000000000000000 ) ) ;
#25631=ADVANCED_FACE ( 'NONE', ( #19082 ), #26385, .T. ) ;
#25632=TOROIDAL_SURFACE ( 'NONE', #6245, 0.5610236220472440971, 0.1003937007874015908 ) ;
#25645=ORIENTED_EDGE ( 'NONE', *, *, #14701, .F. ) ;
#25651=ORIENTED_EDGE ( 'NONE', *, *, #8711, .F. ) ;
#25652=DIRECTION ( 'NONE',  ( -0.6427876096865396960, -0.7660444431189776804, 0.000000000000000000 ) ) ;
#25659=TOROIDAL_SURFACE ( 'NONE', #13455, 0.5610236220472440971, 0.1003937007874015908 ) ;
#25691=VERTEX_POINT ( 'NONE', #15294 ) ;
#25738=CIRCLE ( 'NONE', #22113, 0.1003937007874015908 ) ;
#25754=CARTESIAN_POINT ( 'NONE',  ( 0.4339912984563291110, -0.2498791196563492356, 0.09685039370078740717 ) ) ;
#25788=CARTESIAN_POINT ( 'NONE',  ( -0.5572789388079989470, -0.3225230913464889881, 0.2359405056214250451 ) ) ;
#25799=AXIS2_PLACEMENT_3D ( 'NONE', #2396, #13279, #17383 ) ;
#25808=CARTESIAN_POINT ( 'NONE',  ( 0.4690668203920866919, 0.08212126673946905375, 0.1212655228496834631 ) ) ;
#25825=VERTEX_POINT ( 'NONE', #7070 ) ;
#25829=ORIENTED_EDGE ( 'NONE', *, *, #10300, .F. ) ;
#25841=CARTESIAN_POINT ( 'NONE',  ( 0.0002199787722625489263, 0.6212598425196850238, 0.2574827755769818483 ) ) ;
#25854=DIRECTION ( 'NONE',  ( 1.000000000000000000, 0.000000000000000000, 0.000000000000000000 ) ) ;
#25862=DIRECTION ( 'NONE',  ( 0.000000000000000000, 0.000000000000000000, 1.000000000000000000 ) ) ;
#25865=CARTESIAN_POINT ( 'NONE',  ( 0.3056525133794348315, 0.3651631491574845456, 0.2330651858023968237 ) ) ;
#25873=DIRECTION ( 'NONE',  ( 0.000000000000000000, 1.000000000000000000, 0.000000000000000000 ) ) ;
#25906=CARTESIAN_POINT ( 'NONE',  ( 0.000000000000000000, 0.000000000000000000, 0.2574803149606298969 ) ) ;
#25912=TOROIDAL_SURFACE ( 'NONE', #13713, 0.5610236220472440971, 0.1003937007874015908 ) ;
#25926=DIRECTION ( 'NONE',  ( 1.000000000000000000, 0.000000000000000000, 0.000000000000000000 ) ) ;
#25939=CARTESIAN_POINT ( 'NONE',  ( -0.6117833106356003192, 0.1080972763116098551, 0.2574827755769819038 ) ) ;
#25942=CARTESIAN_POINT ( 'NONE',  ( 0.000000000000000000, 0.000000000000000000, 0.1771653543307086520 ) ) ;
#25944=ORIENTED_EDGE ( 'NONE', *, *, #23690, .T. ) ;
#25957=ORIENTED_EDGE ( 'NONE', *, *, #18480, .F. ) ;
#25958=B_SPLINE_CURVE_WITH_KNOTS ( 'NONE', 3,
 ( #24814, #11969, #14086, #22703, #25239, #5763 ),
 .UNSPECIFIED., .F., .F.,
 ( 4, 2, 4 ),
 ( 0.9359046326925629655, 0.9375808709372029925, 0.9392571091818440188 ),
 .UNSPECIFIED. ) ;
#25981=AXIS2_PLACEMENT_3D ( 'NONE', #11712, #20335, #18188 ) ;
#26006=VECTOR ( 'NONE', #3135, 39.37007874015748143 ) ;
#26016=ORIENTED_EDGE ( 'NONE', *, *, #7300, .F. ) ;
#26017=CARTESIAN_POINT ( 'NONE',  ( 0.000000000000000000, 0.000000000000000000, 0.2574803149606298969 ) ) ;
#26022=EDGE_CURVE ( 'NONE', #23891, #18882, #9717, .T. ) ;
#26032=CARTESIAN_POINT ( 'NONE',  ( 0.000000000000000000, 0.000000000000000000, 0.1771653543307086520 ) ) ;
#26033=CARTESIAN_POINT ( 'NONE',  ( -0.4537304931026616139, 0.07942646906834205378, 0.1771653543307086243 ) ) ;
#26034=CARTESIAN_POINT ( 'NONE',  ( -0.3990005999895763766, 0.4761957181734953193, 0.2574819594177531479 ) ) ;
#26054=ORIENTED_EDGE ( 'NONE', *, *, #4377, .T. ) ;
#26055=FACE_OUTER_BOUND ( 'NONE', #1775, .T. ) ;
#26095=ORIENTED_EDGE ( 'NONE', *, *, #1911, .F. ) ;
#26111=AXIS2_PLACEMENT_3D ( 'NONE', #17179, #2829, #26431 ) ;
#26115=CIRCLE ( 'NONE', #5366, 0.4606299212598425341 ) ;
#26119=EDGE_CURVE ( 'NONE', #14713, #12635, #20080, .T. ) ;
#26128=CARTESIAN_POINT ( 'NONE',  ( -0.1589886963207482462, -0.4351482077919938685, 0.1494804571204739196 ) ) ;
#26130=CARTESIAN_POINT ( 'NONE',  ( 0.7165354330708662012, 0.000000000000000000, 0.3543307086614173040 ) ) ;
#26165=ORIENTED_EDGE ( 'NONE', *, *, #21415, .T. ) ;
#26173=B_SPLINE_CURVE_WITH_KNOTS ( 'NONE', 3,
 ( #26450, #21684, #11350, #19967, #24338, #7113, #17573, #13185, #15736, #2311 ),
 .UNSPECIFIED., .F., .F.,
 ( 4, 2, 2, 2, 4 ),
 ( 0.000000000000000000, 0.2500000000000000000, 0.5000000000000000000, 0.7500000000000000000, 1.000000000000000000 ),
 .UNSPECIFIED. ) ;
#26181=FACE_OUTER_BOUND ( 'NONE', #17775, .T. ) ;
#26183=CARTESIAN_POINT ( 'NONE',  ( 0.000000000000000000, 0.6212598425196850238, 0.3543307086614173040 ) ) ;
#26186=EDGE_CURVE ( 'NONE', #17148, #14935, #6038, .T. ) ;
#26188=CARTESIAN_POINT ( 'NONE',  ( -0.1707210962531915677, -0.4707890492249701131, 0.2574803149606298969 ) ) ;
#26190=CARTESIAN_POINT ( 'NONE',  ( 0.3990005999895235855, 0.4761957181735393396, 0.2574819594177527593 ) ) ;
#26206=EDGE_CURVE ( 'NONE', #12846, #8161, #12883, .T. ) ;
#26217=DIRECTION ( 'NONE',  ( 0.000000000000000000, 0.000000000000000000, 1.000000000000000000 ) ) ;
#26234=DIRECTION ( 'NONE',  ( -0.9396926207859083169, 0.3420201433256692125, 0.000000000000000000 ) ) ;
#26253=CARTESIAN_POINT ( 'NONE',  ( 0.4210617728738614285, -0.2437762437824630424, 0.1075369453634683753 ) ) ;
#26259=B_SPLINE_CURVE_WITH_KNOTS ( 'NONE', 3,
 ( #27667, #22122, #24376, #5018 ),
 .UNSPECIFIED., .F., .F.,
 ( 4, 4 ),
 ( 0.3108507187342950395, 0.3125269569790670721 ),
 .UNSPECIFIED. ) ;
#26260=FACE_OUTER_BOUND ( 'NONE', #19186, .T. ) ;
#26269=CARTESIAN_POINT ( 'NONE',  ( 0.6212598425196850238, 0.000000000000000000, 0.2574803149606298969 ) ) ;
#26277=ORIENTED_EDGE ( 'NONE', *, *, #27539, .T. ) ;
#26282=FACE_OUTER_BOUND ( 'NONE', #15411, .T. ) ;
#26307=ADVANCED_FACE ( 'NONE', ( #3079 ), #13346, .F. ) ;
#26314=AXIS2_PLACEMENT_3D ( 'NONE', #22267, #2899, #24802 ) ;
#26319=CARTESIAN_POINT ( 'NONE',  ( 0.4256740239341992305, 0.5062356173701832995, 0.1926811207699622719 ) ) ;
#26320=TOROIDAL_SURFACE ( 'NONE', #21814, 0.5610236220472440971, 0.1003937007874015908 ) ;
#26325=EDGE_LOOP ( 'NONE', ( #18881, #14868 ) ) ;
#26338=CARTESIAN_POINT ( 'NONE',  ( 0.000000000000000000, 0.000000000000000000, 0.09685039370078740717 ) ) ;
#26339=CARTESIAN_POINT ( 'NONE',  ( 0.6239291699153675097, 0.1106940470467558946, 0.2481708550953252990 ) ) ;
#26344=VECTOR ( 'NONE', #3399, 39.37007874015748143 ) ;
#26356=AXIS2_PLACEMENT_3D ( 'NONE', #16675, #24856, #14579 ) ;
#26370=CIRCLE ( 'NONE', #23249, 0.5007874015748031704 ) ;
#26385=TOROIDAL_SURFACE ( 'NONE', #7006, 0.7165354330708662012, 0.01181102362204724393 ) ;
#26393=VERTEX_POINT ( 'NONE', #21374 ) ;
#26399=CARTESIAN_POINT ( 'NONE',  ( 0.4537304931026562849, 0.07942646906837143306, 0.1771653543307087630 ) ) ;
#26400=EDGE_CURVE ( 'NONE', #8161, #10058, #5215, .T. ) ;
#26416=CARTESIAN_POINT ( 'NONE',  ( -0.0005939837304750000086, 0.5007870493127504208, 0.2574803149606298969 ) ) ;
#26431=DIRECTION ( 'NONE',  ( 0.1736481776669299981, -0.9848077530122081313, 0.000000000000000000 ) ) ;
#26432=CARTESIAN_POINT ( 'NONE',  ( 0.000000000000000000, 0.000000000000000000, 0.1771653543307086520 ) ) ;
#26433=ORIENTED_EDGE ( 'NONE', *, *, #20354, .T. ) ;
#26437=CARTESIAN_POINT ( 'NONE',  ( 0.000000000000000000, 0.000000000000000000, 0.1771653543307086520 ) ) ;
#26441=CARTESIAN_POINT ( 'NONE',  ( -0.4535326485287287657, 0.08054850140359764987, 0.1771653543307088186 ) ) ;
#26446=CARTESIAN_POINT ( 'NONE',  ( 0.1716509673353401599, -0.4704508543867079173, 0.2574819596263889787 ) ) ;
#26448=CARTESIAN_POINT ( 'NONE',  ( 0.3215969074633125979, 0.3838795254899315390, 0.2574819596263889787 ) ) ;
#26450=CARTESIAN_POINT ( 'NONE',  ( -0.0006615832606325197825, 0.6212594902576319411, 0.09685039370078740717 ) ) ;
#26451=EDGE_CURVE ( 'NONE', #11735, #1869, #15155, .T. ) ;
#26457=ORIENTED_EDGE ( 'NONE', *, *, #18967, .F. ) ;
#26463=CARTESIAN_POINT ( 'NONE',  ( 0.0005696707463081693290, 0.4606295689977896735, 0.1639447408819529051 ) ) ;
#26473=CARTESIAN_POINT ( 'NONE',  ( 0.2965233727166233790, 0.3524965443697388734, 0.1771653543307087630 ) ) ;
#26505=FACE_OUTER_BOUND ( 'NONE', #24933, .T. ) ;
#26511=AXIS2_PLACEMENT_3D ( 'NONE', #195, #2261, #8763 ) ;
#26517=ORIENTED_EDGE ( 'NONE', *, *, #10870, .T. ) ;
#26526=ORIENTED_EDGE ( 'NONE', *, *, #20377, .T. ) ;
#26528=DIRECTION ( 'NONE',  ( 0.000000000000000000, -1.000000000000000000, 0.000000000000000000 ) ) ;
#26529=CARTESIAN_POINT ( 'NONE',  ( 0.5610236220472440971, 0.000000000000000000, 0.1771653543307086520 ) ) ;
#26530=CARTESIAN_POINT ( 'NONE',  ( -0.0002199787722797783896, 0.6212598425196852459, 0.09684793308443542803 ) ) ;
#26549=VERTEX_POINT ( 'NONE', #20070 ) ;
#26553=VERTEX_POINT ( 'NONE', #9461 ) ;
#26562=CARTESIAN_POINT ( 'NONE',  ( 0.4335958738490826581, -0.2505647196907697105, 0.2574827755769819038 ) ) ;
#26575=CARTESIAN_POINT ( 'NONE',  ( 0.6118978891064095205, 0.1074467966294586629, 0.2574819594177531479 ) ) ;
#26578=CARTESIAN_POINT ( 'NONE',  ( -0.3606190329934327310, 0.4297690281277732338, 0.1771653543307086520 ) ) ;
#26583=PLANE ( 'NONE',  #1374 ) ;
#26586=DIRECTION ( 'NONE',  ( 0.000000000000000000, 0.000000000000000000, -1.000000000000000000 ) ) ;
#26588=CARTESIAN_POINT ( 'NONE',  ( -0.5579526598176230978, -0.3213561723287879368, 0.1183902030406979167 ) ) ;
#26590=SPHERICAL_SURFACE ( 'NONE', #7044, 0.1003956692913385851 ) ;
#26609=CARTESIAN_POINT ( 'NONE',  ( 0.0001974756197917672956, 0.5007874015748032814, 0.09684793308443545579 ) ) ;
#26613=EDGE_CURVE ( 'NONE', #25691, #20032, #26874, .T. ) ;
#26616=AXIS2_PLACEMENT_3D ( 'NONE', #14975, #19616, #27818 ) ;
#26617=ORIENTED_EDGE ( 'NONE', *, *, #2902, .F. ) ;
#26633=ORIENTED_EDGE ( 'NONE', *, *, #6112, .F. ) ;
#26635=CARTESIAN_POINT ( 'NONE',  ( -0.3986320731132244610, -0.2308081338369635804, 0.1771653543307087630 ) ) ;
#26636=ORIENTED_EDGE ( 'NONE', *, *, #23876, .F. ) ;
#26677=CARTESIAN_POINT ( 'NONE',  ( -0.0004405150045870545247, 0.6212597256746517083, 0.09684874924366457249 ) ) ;
#26693=DIRECTION ( 'NONE',  ( 0.000000000000000000, 0.000000000000000000, 1.000000000000000000 ) ) ;
#26710=VERTEX_POINT ( 'NONE', #20916 ) ;
#26727=CARTESIAN_POINT ( 'NONE',  ( 0.1718374205099799101, -0.4703827404237102550, 0.2574803149606298969 ) ) ;
#26730=ADVANCED_FACE ( 'NONE', ( #1417 ), #24626, .F. ) ;
#26736=CARTESIAN_POINT ( 'NONE',  ( -8.919671568592927398E-17, -0.7283464566929134243, 0.3425196850393700809 ) ) ;
#26746=EDGE_CURVE ( 'NONE', #2008, #7423, #21536, .T. ) ;
#26768=TOROIDAL_SURFACE ( 'NONE', #18179, 0.5610236220472440971, 0.1003937007874015908 ) ;
#26796=EDGE_CURVE ( 'NONE', #13188, #24177, #5699, .T. ) ;
#26800=CARTESIAN_POINT ( 'NONE',  ( -0.3995066426835732765, 0.4757712504659606378, 0.09684793308443542803 ) ) ;
#26808=ORIENTED_EDGE ( 'NONE', *, *, #14701, .T. ) ;
#26828=ADVANCED_FACE ( 'NONE', ( #6504 ), #12581, .T. ) ;
#26830=CARTESIAN_POINT ( 'NONE',  ( -0.4133615125884808061, 0.4936731914940779564, 0.1183902030387112697 ) ) ;
#26831=B_SPLINE_CURVE_WITH_KNOTS ( 'NONE', 3,
 ( #24021, #15012, #15150, #4534, #4398, #13004 ),
 .UNSPECIFIED., .F., .F.,
 ( 4, 2, 4 ),
 ( 0.000000000000000000, 0.2500000000000000000, 0.5000000000000000000 ),
 .UNSPECIFIED. ) ;
#26874=CIRCLE ( 'NONE', #12466, 0.01181102362204730985 ) ;
#26875=CARTESIAN_POINT ( 'NONE',  ( -0.3606190329934327310, 0.4297690281277732338, 0.1771653543307086520 ) ) ;
#26906=EDGE_CURVE ( 'NONE', #14713, #22576, #21193, .T. ) ;
#26907=ADVANCED_FACE ( 'NONE', ( #17238 ), #14763, .F. ) ;
#26908=B_SPLINE_CURVE_WITH_KNOTS ( 'NONE', 3,
 ( #27286, #25447, #10321, #12160, #16406, #14159 ),
 .UNSPECIFIED., .F., .F.,
 ( 4, 2, 4 ),
 ( 0.9031406754215579591, 0.9046454396443720514, 0.9061502038671850334 ),
 .UNSPECIFIED. ) ;
#26914=EDGE_CURVE ( 'NONE', #8934, #4649, #2534, .T. ) ;
#26922=EDGE_CURVE ( 'NONE', #24718, #5673, #4781, .T. ) ;
#26937=CARTESIAN_POINT ( 'NONE',  ( 0.000000000000000000, 0.000000000000000000, 0.1771653543307086520 ) ) ;
#26949=CARTESIAN_POINT ( 'NONE',  ( 0.3992017438595159562, -0.2298214351608004746, 0.1771653543307084855 ) ) ;
#26967=ORIENTED_EDGE ( 'NONE', *, *, #23544, .T. ) ;
#26974=CARTESIAN_POINT ( 'NONE',  ( -0.1589886963208103077, -0.4351482077921629554, 0.2048502515415793201 ) ) ;
#26977=CARTESIAN_POINT ( 'NONE',  ( -0.4222761783096392052, 0.5043089796487417731, 0.1461456498289284978 ) ) ;
#26983=AXIS2_PLACEMENT_3D ( 'NONE', #3256, #24598, #24742 ) ;
#26985=CARTESIAN_POINT ( 'NONE',  ( 0.2131049448084480213, -0.5835666837866708700, 0.2574803149606298969 ) ) ;
#26994=B_SPLINE_CURVE_WITH_KNOTS ( 'NONE', 3,
 ( #14452, #18360, #20787, #23062, #27579, #9906, #12162, #18793, #25017, #5684 ),
 .UNSPECIFIED., .F., .F.,
 ( 4, 2, 2, 2, 4 ),
 ( 0.000000000000000000, 0.2500000000000000000, 0.5000000000000000000, 0.7500000000000000000, 1.000000000000000000 ),
 .UNSPECIFIED. ) ;
#27000=ORIENTED_EDGE ( 'NONE', *, *, #23302, .F. ) ;
#27005=DIRECTION ( 'NONE',  ( 0.000000000000000000, 0.000000000000000000, 1.000000000000000000 ) ) ;
#27007=CIRCLE ( 'NONE', #16181, 0.7283464566929134243 ) ;
#27021=CARTESIAN_POINT ( 'NONE',  ( 0.000000000000000000, 0.000000000000000000, 0.2574803149606298969 ) ) ;
#27022=VERTEX_POINT ( 'NONE', #15674 ) ;
#27028=DIRECTION ( 'NONE',  ( -0.6427876096865392519, 0.7660444431189780135, 0.000000000000000000 ) ) ;
#27032=EDGE_LOOP ( 'NONE', ( #26967, #21528, #11909, #16191 ) ) ;
#27036=CARTESIAN_POINT ( 'NONE',  ( 0.000000000000000000, 0.6212598425196850238, -3.278217716535432842E-17 ) ) ;
#27042=DIRECTION ( 'NONE',  ( 1.000000000000000000, 0.000000000000000000, 0.000000000000000000 ) ) ;
#27044=DIRECTION ( 'NONE',  ( 1.000000000000000000, 0.000000000000000000, 0.000000000000000000 ) ) ;
#27087=DIRECTION ( 'NONE',  ( 0.000000000000000000, 0.000000000000000000, 1.000000000000000000 ) ) ;
#27092=DIRECTION ( 'NONE',  ( -0.8660254037844387076, 0.4999999999999998890, 0.000000000000000000 ) ) ;
#27100=CARTESIAN_POINT ( 'NONE',  ( 0.000000000000000000, 0.000000000000000000, 0.1771653543307086520 ) ) ;
#27120=CARTESIAN_POINT ( 'NONE',  ( 0.000000000000000000, 0.000000000000000000, 0.1771653543307086520 ) ) ;
#27121=EDGE_CURVE ( 'NONE', #24230, #17929, #16786, .T. ) ;
#27122=CARTESIAN_POINT ( 'NONE',  ( 0.5383572925355968319, -0.3100567972183901899, 0.09685039370078740717 ) ) ;
#27134=AXIS2_PLACEMENT_3D ( 'NONE', #13686, #566, #18181 ) ;
#27135=AXIS2_PLACEMENT_3D ( 'NONE', #14062, #1074, #13775 ) ;
#27137=CARTESIAN_POINT ( 'NONE',  ( 0.3214446924536846772, 0.3840069416942866742, 0.09685039370078740717 ) ) ;
#27154=CARTESIAN_POINT ( 'NONE',  ( -0.0005939837304750000086, 0.5007870493127504208, 0.09685039370078740717 ) ) ;
#27172=ORIENTED_EDGE ( 'NONE', *, *, #16269, .F. ) ;
#27174=ORIENTED_EDGE ( 'NONE', *, *, #27758, .T. ) ;
#27181=EDGE_CURVE ( 'NONE', #11007, #15797, #12958, .T. ) ;
#27183=CARTESIAN_POINT ( 'NONE',  ( -0.1718374205099799101, -0.4703827404237102550, 0.2574803149606298969 ) ) ;
#27190=CARTESIAN_POINT ( 'NONE',  ( -0.2118615749922468650, -0.5840192333899535404, 0.2574803149606298969 ) ) ;
#27201=ORIENTED_EDGE ( 'NONE', *, *, #10554, .T. ) ;
#27202=( LENGTH_UNIT ( ) NAMED_UNIT ( * ) SI_UNIT ( $, .METRE. ) ) ;
#27203=AXIS2_PLACEMENT_3D ( 'NONE', #11211, #2588, #15610 ) ;
#27204=ORIENTED_EDGE ( 'NONE', *, *, #21337, .T. ) ;
#27213=ORIENTED_EDGE ( 'NONE', *, *, #14708, .T. ) ;
#27215=DIRECTION ( 'NONE',  ( 0.3420201433256691570, -0.9396926207859082059, 0.000000000000000000 ) ) ;
#27230=AXIS2_PLACEMENT_3D ( 'NONE', #6083, #12696, #10290 ) ;
#27231=DIRECTION ( 'NONE',  ( 0.000000000000000000, 0.000000000000000000, 1.000000000000000000 ) ) ;
#27249=VERTEX_POINT ( 'NONE', #11119 ) ;
#27264=CARTESIAN_POINT ( 'NONE',  ( -0.7165354330708662012, 8.847349907225958695E-17, -3.278217716535432842E-17 ) ) ;
#27271=ORIENTED_EDGE ( 'NONE', *, *, #7627, .F. ) ;
#27286=CARTESIAN_POINT ( 'NONE',  ( -0.1718374205099799101, -0.4703827404237102550, 0.2574803149606298969 ) ) ;
#27287=DIRECTION ( 'NONE',  ( 0.1736481776669313026, 0.9848077530122077983, 0.000000000000000000 ) ) ;
#27294=EDGE_CURVE ( 'NONE', #6009, #13528, #11717, .T. ) ;
#27297=ORIENTED_EDGE ( 'NONE', *, *, #17648, .T. ) ;
#27324=ADVANCED_FACE ( 'NONE', ( #24216 ), #5722, .F. ) ;
#27342=PRESENTATION_STYLE_ASSIGNMENT (( #20700 ) ) ;
#27352=CARTESIAN_POINT ( 'NONE',  ( -0.5724622793729822190, -0.3313001865996386686, 0.1616495878883337511 ) ) ;
#27363=FACE_BOUND ( 'NONE', #12148, .T. ) ;
#27375=CARTESIAN_POINT ( 'NONE',  ( 0.3223547283257516272, 0.3832433309296771617, 0.2574803149606298969 ) ) ;
#27378=ADVANCED_FACE ( 'NONE', ( #13198, #15204 ), #8955, .T. ) ;
#27385=CARTESIAN_POINT ( 'NONE',  ( 0.4535326485287339282, 0.08054850140356757671, 0.1771653543307084855 ) ) ;
#27390=ORIENTED_EDGE ( 'NONE', *, *, #705, .T. ) ;
#27392=ORIENTED_EDGE ( 'NONE', *, *, #4810, .T. ) ;
#27395=B_SPLINE_CURVE_WITH_KNOTS ( 'NONE', 3,
 ( #16660, #12270, #14416, #1393, #19044, #21031 ),
 .UNSPECIFIED., .F., .F.,
 ( 4, 2, 4 ),
 ( 0.3108507187342960387, 0.3125269569790670166, 0.3142031952238389936 ),
 .UNSPECIFIED. ) ;
#27401=CARTESIAN_POINT ( 'NONE',  ( -0.4333973147258542991, -0.2509079296564011852, 0.2574803149606298969 ) ) ;
#27423=CARTESIAN_POINT ( 'NONE',  ( -0.2243259791915123424, -0.6183223858009434526, 0.2081850588310771299 ) ) ;
#27430=CARTESIAN_POINT ( 'NONE',  ( -0.1570092758121683085, -0.4330450457732859526, 0.1639447408239428638 ) ) ;
#27456=ORIENTED_EDGE ( 'NONE', *, *, #4830, .T. ) ;
#27462=ADVANCED_FACE ( 'NONE', ( #9932 ), #20613, .F. ) ;
#27463=VERTEX_POINT ( 'NONE', #27183 ) ;
#27471=AXIS2_PLACEMENT_3D ( 'NONE', #10854, #19469, #8734 ) ;
#27478=EDGE_LOOP ( 'NONE', ( #15055, #9050, #12254, #4246, #12400, #5461 ) ) ;
#27482=CARTESIAN_POINT ( 'NONE',  ( 0.3988311005573134116, 0.4763376377694984454, 0.09685039370078740717 ) ) ;
#27487=CARTESIAN_POINT ( 'NONE',  ( 0.3986320731132086959, -0.2308081338369904478, 0.1771653543307089018 ) ) ;
#27488=CARTESIAN_POINT ( 'NONE',  ( 0.2173565190940987546, -0.5952284643178856749, 0.2481708550929211665 ) ) ;
#27489=VERTEX_POINT ( 'NONE', #11775 ) ;
#27502=FACE_OUTER_BOUND ( 'NONE', #14276, .T. ) ;
#27512=EDGE_CURVE ( 'NONE', #8934, #12846, #9011, .T. ) ;
#27514=CARTESIAN_POINT ( 'NONE',  ( 0.0006812437162516955368, 0.6577569867585544294, 0.2081850588313099992 ) ) ;
#27519=CARTESIAN_POINT ( 'NONE',  ( 0.000000000000000000, 0.000000000000000000, 0.1771653543307086520 ) ) ;
#27521=EDGE_CURVE ( 'NONE', #23101, #833, #4663, .T. ) ;
#27524=CARTESIAN_POINT ( 'NONE',  ( -0.2131049448083992270, -0.5835666837866889667, 0.09685039370078740717 ) ) ;
#27539=EDGE_CURVE ( 'NONE', #2920, #6078, #3915, .T. ) ;
#27565=CARTESIAN_POINT ( 'NONE',  ( 0.4930758245789425009, 0.08754571829529310401, 0.09685039370078740717 ) ) ;
#27579=CARTESIAN_POINT ( 'NONE',  ( -0.6514872030408946912, 0.1141809932447457321, 0.1616495878811869680 ) ) ;
#27580=CARTESIAN_POINT ( 'NONE',  ( 0.5376957092749897749, -0.3112026930391976753, 0.2574803149606298969 ) ) ;
#27593=AXIS2_PLACEMENT_3D ( 'NONE', #18822, #12062, #7969 ) ;
#27598=FACE_OUTER_BOUND ( 'NONE', #8048, .T. ) ;
#27629=CARTESIAN_POINT ( 'NONE',  ( 0.2256062985769322349, -0.6178563876516726117, 0.1461456498233222601 ) ) ;
#27630=ADVANCED_FACE ( 'NONE', ( #10070 ), #7977, .F. ) ;
#27635=CIRCLE ( 'NONE', #17267, 0.6212598425196850238 ) ;
#27642=ORIENTED_EDGE ( 'NONE', *, *, #3593, .T. ) ;
#27644=CARTESIAN_POINT ( 'NONE',  ( -0.7165354330708662012, 8.775028245858987528E-17, 0.01181102362204724393 ) ) ;
#27650=CARTESIAN_POINT ( 'NONE',  ( 0.6239291699165746552, 0.1106940470469692378, 0.1061598535670113391 ) ) ;
#27652=CARTESIAN_POINT ( 'NONE',  ( 0.0006681923949035713933, 0.6336721034125017971, 0.1061598535669395216 ) ) ;
#27657=ORIENTED_EDGE ( 'NONE', *, *, #23992, .F. ) ;
#27667=CARTESIAN_POINT ( 'NONE',  ( 0.0006615832606325197825, 0.6212594902576319411, 0.09685039370078740717 ) ) ;
#27683=VERTEX_POINT ( 'NONE', #23620 ) ;
#27695=EDGE_CURVE ( 'NONE', #1869, #6477, #11028, .T. ) ;
#27701=CIRCLE ( 'NONE', #1977, 0.5007874015748031704 ) ;
#27704=DIRECTION ( 'NONE',  ( 0.000000000000000000, 1.000000000000000000, 0.000000000000000000 ) ) ;
#27710=B_SPLINE_CURVE_WITH_KNOTS ( 'NONE', 3,
 ( #16908, #6314, #12522, #21140 ),
 .UNSPECIFIED., .F., .F.,
 ( 4, 4 ),
 ( 0.9031406754215589583, 0.9046454396443728285 ),
 .UNSPECIFIED. ) ;
#27714=CARTESIAN_POINT ( 'NONE',  ( 0.4792483803807430776, 0.08390985360578698260, 0.2467937633143996445 ) ) ;
#27720=DIRECTION ( 'NONE',  ( 0.000000000000000000, 0.000000000000000000, 1.000000000000000000 ) ) ;
#27726=CIRCLE ( 'NONE', #2855, 0.01181102362204724046 ) ;
#27731=ORIENTED_EDGE ( 'NONE', *, *, #11322, .T. ) ;
#27751=CARTESIAN_POINT ( 'NONE',  ( 0.000000000000000000, 0.3937007874015748254, 0.3425196850393700809 ) ) ;
#27758=EDGE_CURVE ( 'NONE', #25113, #23041, #9662, .T. ) ;
#27765=CARTESIAN_POINT ( 'NONE',  ( -0.2956505864974143805, 0.3532288989643735944, 0.1639447408836617603 ) ) ;
#27769=CARTESIAN_POINT ( 'NONE',  ( 0.3986320731132085848, -0.2308081338369909197, 0.1903859677802542949 ) ) ;
#27798=VERTEX_POINT ( 'NONE', #7353 ) ;
#27818=DIRECTION ( 'NONE',  ( 0.000000000000000000, 1.000000000000000000, 0.000000000000000000 ) ) ;
#27837=EDGE_LOOP ( 'NONE', ( #10844, #6713, #12594, #23847 ) ) ;
#27864=CARTESIAN_POINT ( 'NONE',  ( 0.0005710523241086142487, 0.4632828964888820455, 0.2048502514553257048 ) ) ;
#27878=CARTESIAN_POINT ( 'NONE',  ( -0.4858607088160732390, -0.2805118110236220486, 0.2775610236220472093 ) ) ;
ENDSEC;
END-ISO-10303-21;
